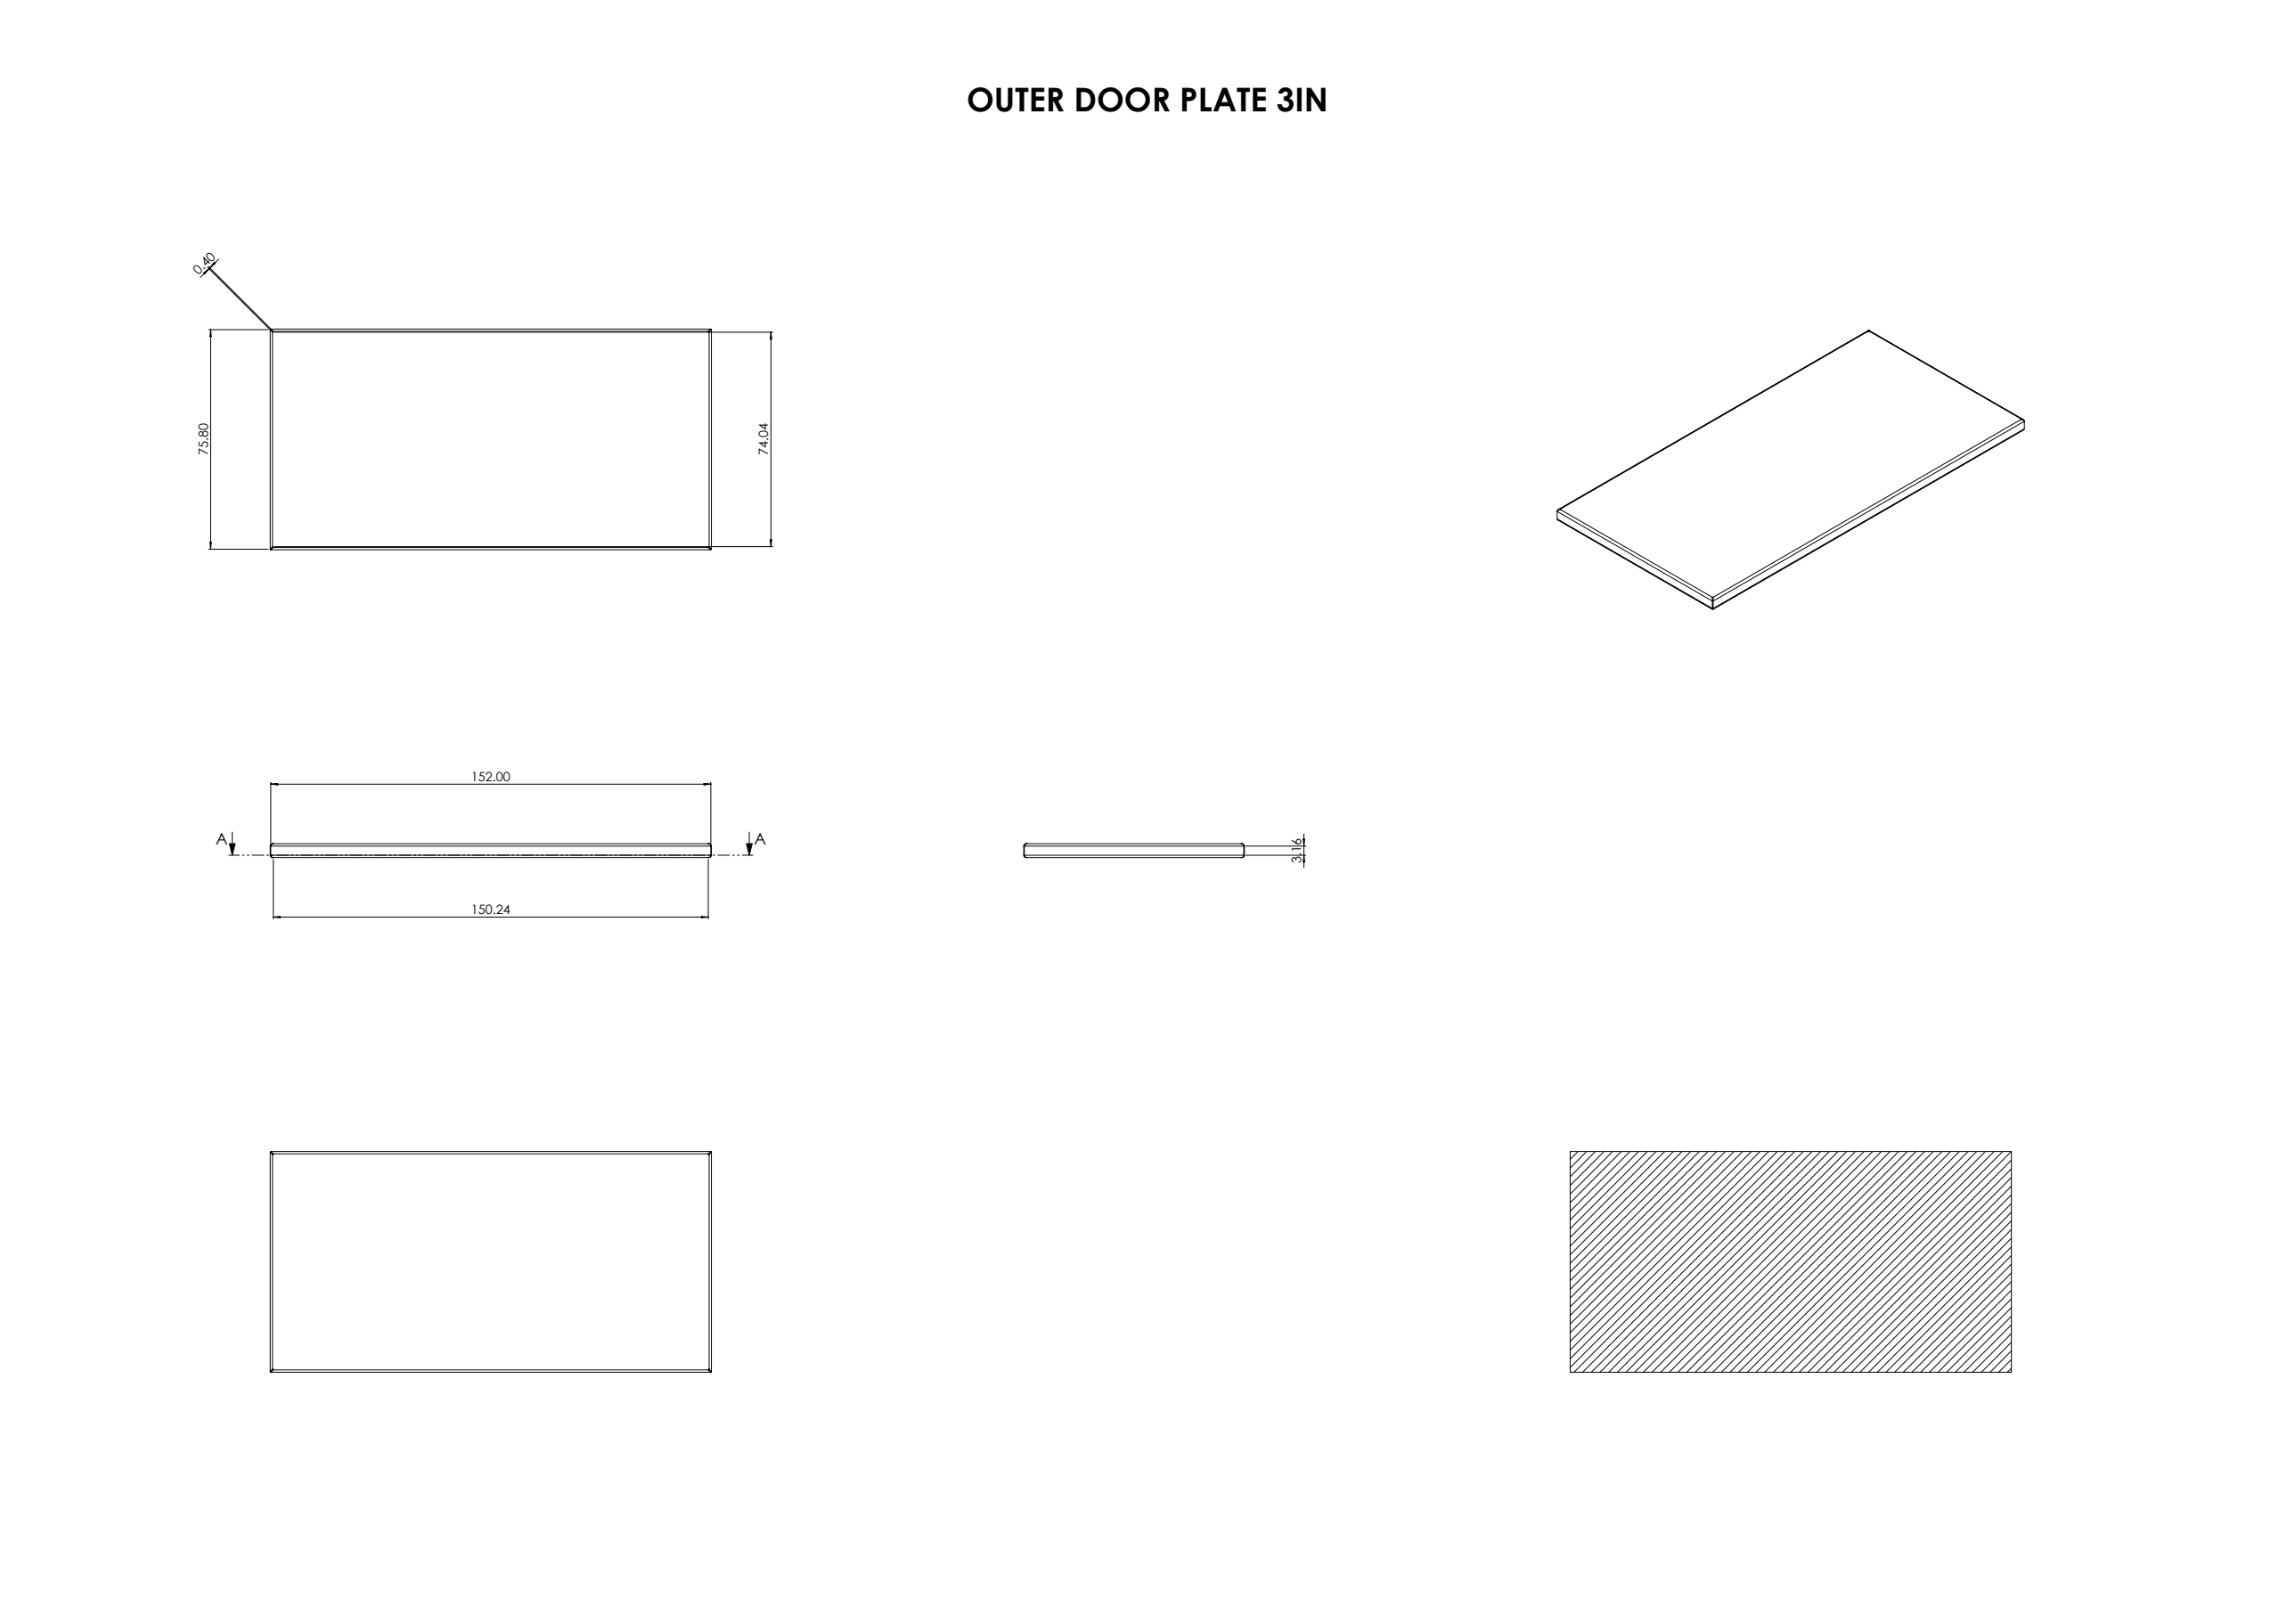
ISO-10303-21;
HEADER;
/* Generated by software containing ST-Developer
 * from STEP Tools, Inc. (www.steptools.com) 
 */

FILE_DESCRIPTION(
/* description */ (''),
/* implementation_level */ '2;1');

FILE_NAME(
/* name */ '03_Outer_Door_Plate_3in.step',
/* time_stamp */ '2026-10-25T01:30:15-07:00',
/* author */ (''),
/* organization */ (''),
/* preprocessor_version */ 'ST-DEVELOPER v20.2',
/* originating_system */ 'Autodesk Translation Framework v15.15.0.0',
/* authorisation */ '');

FILE_SCHEMA (('AUTOMOTIVE_DESIGN { 1 0 10303 214 3 1 1 }'));
ENDSEC;

DATA;
#10=MECHANICAL_DESIGN_GEOMETRIC_PRESENTATION_REPRESENTATION('',(#565),#32309);
#152=B_SPLINE_CURVE_WITH_KNOTS('',3,(#20657,#20658,#20659,#20660,#20661,
#20662,#20663,#20664,#20665,#20666,#20667,#20668,#20669,#20670,#20671,#20672,
#20673,#20674,#20675,#20676,#20677,#20678,#20679,#20680,#20681,#20682,#20683,
#20684,#20685,#20686,#20687,#20688,#20689,#20690,#20691,#20692,#20693,#20694,
#20695,#20696,#20697,#20698,#20699,#20700,#20701,#20702),.UNSPECIFIED.,
 .F.,.F.,(4,3,3,3,3,3,3,3,3,3,3,3,3,3,3,4),(0.,0.0572017311997787,0.120330894890366,
0.190833525217158,0.280000607595836,0.370000531646356,0.437396979142466,
0.498588004587218,0.56260087810271,0.634065239675333,0.727489847564673,
0.803842080660462,0.870326860442866,0.931777978459012,0.988871097354878,
1.),.UNSPECIFIED.);
#153=B_SPLINE_CURVE_WITH_KNOTS('',3,(#20704,#20705,#20706,#20707),
 .UNSPECIFIED.,.F.,.F.,(4,4),(0.,1.),.UNSPECIFIED.);
#154=B_SPLINE_CURVE_WITH_KNOTS('',3,(#20709,#20710,#20711,#20712,#20713,
#20714,#20715,#20716,#20717,#20718,#20719,#20720,#20721,#20722,#20723,#20724,
#20725,#20726,#20727,#20728,#20729,#20730,#20731,#20732,#20733,#20734,#20735,
#20736,#20737,#20738,#20739,#20740,#20741,#20742,#20743,#20744,#20745,#20746,
#20747,#20748,#20749,#20750,#20751,#20752,#20753,#20754),.UNSPECIFIED.,
 .F.,.F.,(4,3,3,3,3,3,3,3,3,3,3,3,3,3,3,4),(0.,0.0572030252319241,0.12033380234495,
0.190838689074404,0.28001183745251,0.370010357770946,0.43740667017455,0.498598114868611,
0.562610573399873,0.634075370124963,0.727505599815991,0.803852814389783,
0.870334971805663,0.931784146691265,0.988875797348581,1.),.UNSPECIFIED.);
#155=B_SPLINE_CURVE_WITH_KNOTS('',3,(#20782,#20783,#20784,#20785,#20786,
#20787,#20788,#20789,#20790,#20791,#20792,#20793,#20794,#20795,#20796,#20797,
#20798,#20799,#20800,#20801,#20802,#20803,#20804,#20805,#20806,#20807,#20808,
#20809,#20810,#20811,#20812,#20813,#20814,#20815,#20816,#20817,#20818,#20819,
#20820,#20821,#20822,#20823,#20824,#20825,#20826,#20827),.UNSPECIFIED.,
 .F.,.F.,(4,3,3,3,3,3,3,3,3,3,3,3,3,3,3,4),(0.,0.0572017311995356,0.120330894891212,
0.190833525222983,0.280000607602918,0.370000531652553,0.437396979149437,
0.498588004587769,0.562600878102254,0.634065239673979,0.727489847577867,
0.803842080671477,0.870326860452954,0.931777978465078,0.988871097360322,
1.),.UNSPECIFIED.);
#156=B_SPLINE_CURVE_WITH_KNOTS('',3,(#20829,#20830,#20831,#20832),
 .UNSPECIFIED.,.F.,.F.,(4,4),(0.,1.),.UNSPECIFIED.);
#157=B_SPLINE_CURVE_WITH_KNOTS('',3,(#20834,#20835,#20836,#20837,#20838,
#20839,#20840,#20841,#20842,#20843,#20844,#20845,#20846,#20847,#20848,#20849,
#20850,#20851,#20852,#20853,#20854,#20855,#20856,#20857,#20858,#20859,#20860,
#20861,#20862,#20863,#20864,#20865,#20866,#20867,#20868,#20869,#20870,#20871,
#20872,#20873,#20874,#20875,#20876,#20877,#20878,#20879),.UNSPECIFIED.,
 .F.,.F.,(4,3,3,3,3,3,3,3,3,3,3,3,3,3,3,4),(0.,0.0572030252292159,0.120333802342511,
0.190838689073324,0.280011837455233,0.370010357773329,0.437406670176794,
0.498598114483872,0.562610572991308,0.634075369653291,0.72750559895434,
0.803852813688791,0.870334971170512,0.931784146099022,0.988875796770373,
1.),.UNSPECIFIED.);
#158=B_SPLINE_CURVE_WITH_KNOTS('',3,(#20910,#20911,#20912,#20913,#20914,
#20915,#20916),.UNSPECIFIED.,.F.,.F.,(4,1,1,1,4),(-1.70953476876621,-1.22109626340444,
-0.732657758042664,-0.366328879021332,5.55111512312578E-17),
 .UNSPECIFIED.);
#159=B_SPLINE_CURVE_WITH_KNOTS('',3,(#20919,#20920,#20921,#20922,#20923,
#20924,#20925),.UNSPECIFIED.,.F.,.F.,(4,1,1,1,4),(-5.55111512312578E-17,
0.366328879021332,0.732657758042664,1.22109626340444,1.70953476876621),
 .UNSPECIFIED.);
#160=B_SPLINE_CURVE_WITH_KNOTS('',3,(#20956,#20957,#20958,#20959,#20960,
#20961),.UNSPECIFIED.,.F.,.F.,(4,1,1,4),(-1.70953476876627,-0.976877010723583,
-0.488438505361791,0.),.UNSPECIFIED.);
#161=B_SPLINE_CURVE_WITH_KNOTS('',3,(#20962,#20963,#20964,#20965,#20966,
#20967),.UNSPECIFIED.,.F.,.F.,(4,1,1,4),(0.,0.488438505361791,0.976877010723583,
1.70953476876627),.UNSPECIFIED.);
#162=B_SPLINE_CURVE_WITH_KNOTS('',3,(#20972,#20973,#20974,#20975,#20976,
#20977),.UNSPECIFIED.,.F.,.F.,(4,1,1,4),(-1.70953476876625,-0.976877010723563,
-0.48843850536177,2.22044604925036E-14),.UNSPECIFIED.);
#163=B_SPLINE_CURVE_WITH_KNOTS('',3,(#20979,#20980,#20981,#20982,#20983,
#20984,#20985,#20986,#20987,#20988,#20989,#20990,#20991,#20992,#20993,#20994,
#20995,#20996,#20997,#20998,#20999,#21000,#21001,#21002,#21003,#21004,#21005,
#21006,#21007,#21008,#21009,#21010,#21011,#21012,#21013,#21014,#21015,#21016,
#21017,#21018,#21019,#21020,#21021,#21022,#21023,#21024),.UNSPECIFIED.,
 .F.,.F.,(4,3,3,3,3,3,3,3,3,3,3,3,3,3,3,4),(0.,0.0572017312010985,0.120330894892007,
0.190833525228125,0.28000060761627,0.370000531664237,0.437396979166382,
0.498588004436113,0.562600877944707,0.634065239485818,0.727489847210369,
0.803842080370144,0.870326860183826,0.931777978218593,0.988871097121157,
1.),.UNSPECIFIED.);
#164=B_SPLINE_CURVE_WITH_KNOTS('',3,(#21034,#21035,#21036,#21037,#21038,
#21039,#21040,#21041,#21042,#21043,#21044,#21045,#21046,#21047,#21048,#21049,
#21050,#21051,#21052,#21053,#21054,#21055,#21056,#21057,#21058,#21059,#21060,
#21061,#21062,#21063,#21064,#21065,#21066,#21067,#21068,#21069,#21070,#21071,
#21072,#21073,#21074,#21075,#21076,#21077,#21078,#21079),.UNSPECIFIED.,
 .F.,.F.,(4,3,3,3,3,3,3,3,3,3,3,3,3,3,3,4),(0.,0.0572030252297135,0.120333802345235,
0.19083868907026,0.280011837447865,0.370010357766881,0.437406670170065,
0.498598115100775,0.562610573648761,0.634075370412809,0.727505600383724,
0.803852814849948,0.870334972221295,0.931784147083444,0.988875797723589,
1.),.UNSPECIFIED.);
#165=B_SPLINE_CURVE_WITH_KNOTS('',3,(#21080,#21081,#21082,#21083,#21084,
#21085),.UNSPECIFIED.,.F.,.F.,(4,1,1,4),(-2.2204460492503E-14,0.488438505361761,
0.976877010723545,1.70953476876622),.UNSPECIFIED.);
#166=B_SPLINE_CURVE_WITH_KNOTS('',3,(#21123,#21124,#21125,#21126),
 .UNSPECIFIED.,.F.,.F.,(4,4),(0.,1.),.UNSPECIFIED.);
#167=B_SPLINE_CURVE_WITH_KNOTS('',3,(#21128,#21129,#21130,#21131,#21132,
#21133,#21134,#21135,#21136,#21137,#21138,#21139,#21140,#21141,#21142,#21143,
#21144,#21145,#21146,#21147,#21148,#21149,#21150,#21151,#21152,#21153,#21154,
#21155,#21156,#21157,#21158,#21159,#21160,#21161,#21162,#21163,#21164,#21165,
#21166,#21167,#21168,#21169,#21170,#21171,#21172,#21173),.UNSPECIFIED.,
 .F.,.F.,(4,3,3,3,3,3,3,3,3,3,3,3,3,3,3,4),(0.,0.0572030252310299,0.120333802344518,
0.190838689075309,0.280011837457742,0.370010357775524,0.437406670179767,
0.498598114793286,0.562610573319674,0.634075370032691,0.727505599642952,
0.803852814249658,0.870334971678365,0.931784146571623,0.988875797229984,
1.),.UNSPECIFIED.);
#168=B_SPLINE_CURVE_WITH_KNOTS('',3,(#21200,#21201,#21202,#21203,#21204,
#21205,#21206,#21207,#21208,#21209,#21210,#21211,#21212,#21213,#21214,#21215,
#21216,#21217,#21218,#21219,#21220,#21221,#21222,#21223,#21224,#21225,#21226,
#21227,#21228,#21229,#21230,#21231,#21232,#21233,#21234,#21235,#21236,#21237,
#21238,#21239,#21240,#21241,#21242,#21243,#21244,#21245),.UNSPECIFIED.,
 .F.,.F.,(4,3,3,3,3,3,3,3,3,3,3,3,3,3,3,4),(0.,0.0572017311978579,0.120330894888584,
0.190833525218063,0.280000607593651,0.370000531644445,0.437396979144834,
0.498588004278573,0.562600877772937,0.634065239292226,0.727489846889499,
0.803842080110613,0.87032685994332,0.931777977987771,0.988871096896156,
1.),.UNSPECIFIED.);
#169=B_SPLINE_CURVE_WITH_KNOTS('',3,(#21246,#21247,#21248,#21249),
 .UNSPECIFIED.,.F.,.F.,(4,4),(0.,1.),.UNSPECIFIED.);
#170=B_SPLINE_CURVE_WITH_KNOTS('',3,(#21275,#21276,#21277,#21278,#21279,
#21280),.UNSPECIFIED.,.F.,.F.,(4,1,1,4),(-1.70953476876622,-0.976877010723545,
-0.488438505361761,2.2204460492503E-14),.UNSPECIFIED.);
#171=B_SPLINE_CURVE_WITH_KNOTS('',3,(#21310,#21311,#21312,#21313,#21314,
#21315),.UNSPECIFIED.,.F.,.F.,(4,1,1,4),(-2.22044604925036E-14,0.48843850536177,
0.976877010723563,1.70953476876625),.UNSPECIFIED.);
#172=B_SPLINE_CURVE_WITH_KNOTS('',3,(#21320,#21321,#21322,#21323,#21324,
#21325),.UNSPECIFIED.,.F.,.F.,(4,1,1,4),(-1.70953476876624,-0.976877010723568,
-0.488438505361784,0.),.UNSPECIFIED.);
#173=B_SPLINE_CURVE_WITH_KNOTS('',3,(#21327,#21328,#21329,#21330,#21331,
#21332,#21333,#21334,#21335,#21336,#21337,#21338,#21339,#21340,#21341,#21342,
#21343,#21344,#21345,#21346,#21347,#21348,#21349,#21350,#21351,#21352,#21353,
#21354,#21355,#21356,#21357,#21358,#21359,#21360,#21361,#21362,#21363,#21364,
#21365,#21366,#21367,#21368,#21369,#21370,#21371,#21372),.UNSPECIFIED.,
 .F.,.F.,(4,3,3,3,3,3,3,3,3,3,3,3,3,3,3,4),(0.,0.0572017312023357,0.120330894894396,
0.190833525223119,0.280000607603027,0.370000531652649,0.437396979148621,
0.498588004437818,0.562600877943201,0.634065239490927,0.727489847224149,
0.803842080384343,0.870326860191725,0.931777978222192,0.988871097126222,
1.),.UNSPECIFIED.);
#174=B_SPLINE_CURVE_WITH_KNOTS('',3,(#21380,#21381,#21382,#21383,#21384,
#21385,#21386,#21387,#21388,#21389,#21390,#21391,#21392,#21393,#21394,#21395,
#21396,#21397,#21398,#21399,#21400,#21401,#21402,#21403,#21404,#21405,#21406,
#21407,#21408,#21409,#21410,#21411,#21412,#21413,#21414,#21415,#21416,#21417,
#21418,#21419,#21420,#21421,#21422,#21423,#21424,#21425),.UNSPECIFIED.,
 .F.,.F.,(4,3,3,3,3,3,3,3,3,3,3,3,3,3,3,4),(0.,0.0572030252293332,0.120333802342866,
0.190838689071281,0.280011837454217,0.37001035777244,0.437406670175742,
0.498598114943859,0.562610573478433,0.634075370216571,0.727505599976586,
0.803852814520644,0.870334971919668,0.93178414679375,0.988875797446903,
1.),.UNSPECIFIED.);
#175=B_SPLINE_CURVE_WITH_KNOTS('',3,(#21426,#21427,#21428,#21429,#21430,
#21431),.UNSPECIFIED.,.F.,.F.,(4,1,1,4),(0.,0.488438505361779,0.976877010723558,
1.70953476876623),.UNSPECIFIED.);
#176=B_SPLINE_CURVE_WITH_KNOTS('',3,(#21457,#21458,#21459,#21460,#21461,
#21462,#21463,#21464,#21465,#21466,#21467,#21468,#21469,#21470,#21471,#21472,
#21473,#21474,#21475,#21476,#21477,#21478,#21479,#21480,#21481,#21482,#21483,
#21484,#21485,#21486,#21487,#21488,#21489,#21490,#21491,#21492,#21493,#21494,
#21495,#21496,#21497,#21498,#21499,#21500,#21501,#21502),.UNSPECIFIED.,
 .F.,.F.,(4,3,3,3,3,3,3,3,3,3,3,3,3,3,3,4),(0.,0.0572017311998059,0.120330894890615,
0.190833525219348,0.280000607590358,0.370000531641563,0.437396979142138,
0.498588004431166,0.562600877935177,0.634065239482274,0.72748984722562,
0.803842080384528,0.870326860191735,0.931777978221736,0.988871097122214,
1.),.UNSPECIFIED.);
#177=B_SPLINE_CURVE_WITH_KNOTS('',3,(#21503,#21504,#21505,#21506),
 .UNSPECIFIED.,.F.,.F.,(4,4),(0.,1.),.UNSPECIFIED.);
#178=B_SPLINE_CURVE_WITH_KNOTS('',3,(#21532,#21533,#21534,#21535),
 .UNSPECIFIED.,.F.,.F.,(4,4),(0.,1.),.UNSPECIFIED.);
#179=B_SPLINE_CURVE_WITH_KNOTS('',3,(#21537,#21538,#21539,#21540,#21541,
#21542,#21543,#21544,#21545,#21546,#21547,#21548,#21549,#21550,#21551,#21552,
#21553,#21554,#21555,#21556,#21557,#21558,#21559,#21560,#21561,#21562,#21563,
#21564,#21565,#21566,#21567,#21568,#21569,#21570,#21571,#21572,#21573,#21574,
#21575,#21576,#21577,#21578,#21579,#21580,#21581,#21582),.UNSPECIFIED.,
 .F.,.F.,(4,3,3,3,3,3,3,3,3,3,3,3,3,3,3,4),(0.,0.0572030252325847,0.120333802345704,
0.190838689075859,0.280011837455415,0.370010357773488,0.437406670178867,
0.498598114640677,0.562610573158014,0.634075369846179,0.727505599307959,
0.803852813976729,0.870334971429114,0.931784146336173,0.98887579700217,
1.),.UNSPECIFIED.);
#180=B_SPLINE_CURVE_WITH_KNOTS('',3,(#21610,#21611,#21612,#21613,#21614,
#21615),.UNSPECIFIED.,.F.,.F.,(4,1,1,4),(0.,0.488438505361784,0.976877010723568,
1.70953476876624),.UNSPECIFIED.);
#181=B_SPLINE_CURVE_WITH_KNOTS('',3,(#21644,#21645,#21646,#21647,#21648,
#21649),.UNSPECIFIED.,.F.,.F.,(4,1,1,4),(-1.70953476876623,-0.976877010723558,
-0.488438505361779,0.),.UNSPECIFIED.);
#182=B_SPLINE_CURVE_WITH_KNOTS('',3,(#21675,#21676,#21677,#21678,#21679,
#21680,#21681,#21682,#21683,#21684,#21685,#21686,#21687,#21688,#21689,#21690,
#21691,#21692,#21693,#21694,#21695,#21696,#21697,#21698,#21699,#21700,#21701,
#21702,#21703,#21704,#21705,#21706,#21707,#21708,#21709,#21710,#21711,#21712,
#21713,#21714,#21715,#21716,#21717,#21718,#21719,#21720),.UNSPECIFIED.,
 .F.,.F.,(4,3,3,3,3,3,3,3,3,3,3,3,3,3,3,4),(0.,0.0572017311990066,0.12033089488981,
0.190833525218569,0.280000607592288,0.370000531643252,0.437396979144409,
0.498588004504094,0.562600878013463,0.634065239570545,0.727489847383163,
0.803842080513076,0.87032686030984,0.931777978330153,0.988871097227407,
1.),.UNSPECIFIED.);
#183=B_SPLINE_CURVE_WITH_KNOTS('',3,(#21722,#21723,#21724,#21725),
 .UNSPECIFIED.,.F.,.F.,(4,4),(-1.,0.),.UNSPECIFIED.);
#184=B_SPLINE_CURVE_WITH_KNOTS('',3,(#21726,#21727,#21728,#21729,#21730,
#21731,#21732,#21733,#21734,#21735,#21736,#21737,#21738,#21739,#21740,#21741,
#21742,#21743,#21744,#21745,#21746,#21747,#21748,#21749,#21750,#21751,#21752,
#21753,#21754,#21755,#21756,#21757,#21758,#21759,#21760,#21761,#21762,#21763,
#21764,#21765,#21766,#21767,#21768,#21769,#21770,#21771),.UNSPECIFIED.,
 .F.,.F.,(4,3,3,3,3,3,3,3,3,3,3,3,3,3,3,4),(0.,0.0572030252278138,0.120333802343175,
0.190838689074842,0.280011837442225,0.370010357761947,0.437406670170392,
0.498598115021839,0.562610573562917,0.634075370316736,0.727505600127926,
0.803852814646169,0.87033497203609,0.931784146912104,0.988875797559871,
1.),.UNSPECIFIED.);
#185=B_SPLINE_CURVE_WITH_KNOTS('',3,(#21798,#21799,#21800,#21801,#21802,
#21803,#21804,#21805,#21806,#21807,#21808,#21809,#21810,#21811,#21812,#21813,
#21814,#21815,#21816,#21817,#21818,#21819,#21820,#21821,#21822,#21823,#21824,
#21825,#21826,#21827,#21828,#21829,#21830,#21831,#21832,#21833,#21834,#21835,
#21836,#21837,#21838,#21839,#21840,#21841,#21842,#21843),.UNSPECIFIED.,
 .F.,.F.,(4,3,3,3,3,3,3,3,3,3,3,3,3,3,3,4),(0.,0.0572017312051678,0.12033089489696,
0.190833525228863,0.280000607608025,0.370000531657022,0.437396979162787,
0.498588004452882,0.562600877959885,0.63406523951468,0.727489847284879,
0.803842080435825,0.870326860243776,0.93177797826367,0.988871097172671,
1.),.UNSPECIFIED.);
#186=B_SPLINE_CURVE_WITH_KNOTS('',3,(#21845,#21846,#21847,#21848),
 .UNSPECIFIED.,.F.,.F.,(4,4),(0.,1.),.UNSPECIFIED.);
#187=B_SPLINE_CURVE_WITH_KNOTS('',3,(#21850,#21851,#21852,#21853,#21854,
#21855,#21856,#21857,#21858,#21859,#21860,#21861,#21862,#21863,#21864,#21865,
#21866,#21867,#21868,#21869,#21870,#21871,#21872,#21873,#21874,#21875,#21876,
#21877,#21878,#21879,#21880,#21881,#21882,#21883,#21884,#21885,#21886,#21887,
#21888,#21889,#21890,#21891,#21892,#21893,#21894,#21895),.UNSPECIFIED.,
 .F.,.F.,(4,3,3,3,3,3,3,3,3,3,3,3,3,3,3,4),(0.,0.0572030252315006,0.120333802344992,
0.190838689075267,0.280011837456553,0.370010357774484,0.437406670177093,
0.498598114715166,0.562610573236497,0.634075369937252,0.727505599475578,
0.803852814112987,0.870334971553103,0.931784146452336,0.988875797114711,
1.),.UNSPECIFIED.);
#188=B_SPLINE_CURVE_WITH_KNOTS('',3,(#21922,#21923,#21924,#21925,#21926,
#21927),.UNSPECIFIED.,.F.,.F.,(4,1,1,4),(-1.7095347687662,-0.97687701072354,
-0.488438505361764,1.11854969730985E-14),.UNSPECIFIED.);
#189=B_SPLINE_CURVE_WITH_KNOTS('',3,(#21930,#21931,#21932,#21933,#21934,
#21935),.UNSPECIFIED.,.F.,.F.,(4,1,1,4),(-1.11854969730985E-14,0.488438505361764,
0.97687701072354,1.7095347687662),.UNSPECIFIED.);
#190=B_SPLINE_CURVE_WITH_KNOTS('',3,(#21966,#21967,#21968,#21969,#21970,
#21971),.UNSPECIFIED.,.F.,.F.,(4,1,1,4),(1.43205788482356,2.16471564286623,
2.65315414822802,3.1415926535898),.UNSPECIFIED.);
#191=B_SPLINE_CURVE_WITH_KNOTS('',3,(#21972,#21973,#21974,#21975,#21976,
#21977),.UNSPECIFIED.,.F.,.F.,(4,1,1,4),(-3.1415926535898,-2.65315414822802,
-2.16471564286623,-1.43205788482356),.UNSPECIFIED.);
#431=B_SPLINE_SURFACE_WITH_KNOTS('',3,3,((#20631,#20632,#20633,#20634,#20635,
#20636),(#20637,#20638,#20639,#20640,#20641,#20642),(#20643,#20644,#20645,
#20646,#20647,#20648),(#20649,#20650,#20651,#20652,#20653,#20654)),
 .UNSPECIFIED.,.F.,.F.,.F.,(4,4),(4,1,1,4),(0.,1.),(0.,0.571428571428571,
0.857142857142857,1.),.UNSPECIFIED.);
#432=B_SPLINE_SURFACE_WITH_KNOTS('',3,3,((#20756,#20757,#20758,#20759,#20760,
#20761),(#20762,#20763,#20764,#20765,#20766,#20767),(#20768,#20769,#20770,
#20771,#20772,#20773),(#20774,#20775,#20776,#20777,#20778,#20779)),
 .UNSPECIFIED.,.F.,.F.,.F.,(4,4),(4,1,1,4),(0.,1.),(0.,0.571428571428571,
0.857142857142857,1.),.UNSPECIFIED.);
#433=B_SPLINE_SURFACE_WITH_KNOTS('',3,3,((#20881,#20882,#20883,#20884,#20885,
#20886,#20887),(#20888,#20889,#20890,#20891,#20892,#20893,#20894),(#20895,
#20896,#20897,#20898,#20899,#20900,#20901),(#20902,#20903,#20904,#20905,
#20906,#20907,#20908)),.UNSPECIFIED.,.F.,.F.,.F.,(4,4),(4,1,1,1,4),(0.,
1.),(-1.70953476876621,-1.22109626340444,-0.732657758042664,-0.366328879021332,
5.55111512312578E-17),.UNSPECIFIED.);
#434=B_SPLINE_SURFACE_WITH_KNOTS('',3,3,((#20932,#20933,#20934,#20935,#20936,
#20937),(#20938,#20939,#20940,#20941,#20942,#20943),(#20944,#20945,#20946,
#20947,#20948,#20949),(#20950,#20951,#20952,#20953,#20954,#20955)),
 .UNSPECIFIED.,.F.,.F.,.F.,(4,4),(4,1,1,4),(0.,1.),(-1.70953476876627,-0.976877010723583,
-0.488438505361791,0.),.UNSPECIFIED.);
#435=B_SPLINE_SURFACE_WITH_KNOTS('',3,3,((#21098,#21099,#21100,#21101,#21102,
#21103),(#21104,#21105,#21106,#21107,#21108,#21109),(#21110,#21111,#21112,
#21113,#21114,#21115),(#21116,#21117,#21118,#21119,#21120,#21121)),
 .UNSPECIFIED.,.F.,.F.,.F.,(4,4),(4,1,1,4),(0.,1.),(0.,0.571428571428571,
0.857142857142857,1.),.UNSPECIFIED.);
#436=B_SPLINE_SURFACE_WITH_KNOTS('',3,3,((#21175,#21176,#21177,#21178,#21179,
#21180),(#21181,#21182,#21183,#21184,#21185,#21186),(#21187,#21188,#21189,
#21190,#21191,#21192),(#21193,#21194,#21195,#21196,#21197,#21198)),
 .UNSPECIFIED.,.F.,.F.,.F.,(4,4),(4,1,1,4),(0.,1.),(0.,0.571428571428571,
0.857142857142857,1.),.UNSPECIFIED.);
#437=B_SPLINE_SURFACE_WITH_KNOTS('',3,3,((#21250,#21251,#21252,#21253,#21254,
#21255),(#21256,#21257,#21258,#21259,#21260,#21261),(#21262,#21263,#21264,
#21265,#21266,#21267),(#21268,#21269,#21270,#21271,#21272,#21273)),
 .UNSPECIFIED.,.F.,.F.,.F.,(4,4),(4,1,1,4),(0.,1.),(-1.70953476876622,-0.976877010723545,
-0.488438505361761,2.2204460492503E-14),.UNSPECIFIED.);
#438=B_SPLINE_SURFACE_WITH_KNOTS('',3,3,((#21286,#21287,#21288,#21289,#21290,
#21291),(#21292,#21293,#21294,#21295,#21296,#21297),(#21298,#21299,#21300,
#21301,#21302,#21303),(#21304,#21305,#21306,#21307,#21308,#21309)),
 .UNSPECIFIED.,.F.,.F.,.F.,(4,4),(4,1,1,4),(0.,1.),(-1.70953476876625,-0.976877010723563,
-0.48843850536177,2.22044604925036E-14),.UNSPECIFIED.);
#439=B_SPLINE_SURFACE_WITH_KNOTS('',3,3,((#21432,#21433,#21434,#21435,#21436,
#21437),(#21438,#21439,#21440,#21441,#21442,#21443),(#21444,#21445,#21446,
#21447,#21448,#21449),(#21450,#21451,#21452,#21453,#21454,#21455)),
 .UNSPECIFIED.,.F.,.F.,.F.,(4,4),(4,1,1,4),(0.,1.),(0.,0.571428571428571,
0.857142857142857,1.),.UNSPECIFIED.);
#440=B_SPLINE_SURFACE_WITH_KNOTS('',3,3,((#21507,#21508,#21509,#21510,#21511,
#21512),(#21513,#21514,#21515,#21516,#21517,#21518),(#21519,#21520,#21521,
#21522,#21523,#21524),(#21525,#21526,#21527,#21528,#21529,#21530)),
 .UNSPECIFIED.,.F.,.F.,.F.,(4,4),(4,1,1,4),(0.,1.),(0.,0.571428571428571,
0.857142857142857,1.),.UNSPECIFIED.);
#441=B_SPLINE_SURFACE_WITH_KNOTS('',3,3,((#21584,#21585,#21586,#21587,#21588,
#21589),(#21590,#21591,#21592,#21593,#21594,#21595),(#21596,#21597,#21598,
#21599,#21600,#21601),(#21602,#21603,#21604,#21605,#21606,#21607)),
 .UNSPECIFIED.,.F.,.F.,.F.,(4,4),(4,1,1,4),(0.,1.),(-1.70953476876624,-0.976877010723568,
-0.488438505361784,0.),.UNSPECIFIED.);
#442=B_SPLINE_SURFACE_WITH_KNOTS('',3,3,((#21620,#21621,#21622,#21623,#21624,
#21625),(#21626,#21627,#21628,#21629,#21630,#21631),(#21632,#21633,#21634,
#21635,#21636,#21637),(#21638,#21639,#21640,#21641,#21642,#21643)),
 .UNSPECIFIED.,.F.,.F.,.F.,(4,4),(4,1,1,4),(0.,1.),(-1.70953476876623,-0.976877010723558,
-0.488438505361779,0.),.UNSPECIFIED.);
#443=B_SPLINE_SURFACE_WITH_KNOTS('',3,3,((#21650,#21651,#21652,#21653,#21654,
#21655),(#21656,#21657,#21658,#21659,#21660,#21661),(#21662,#21663,#21664,
#21665,#21666,#21667),(#21668,#21669,#21670,#21671,#21672,#21673)),
 .UNSPECIFIED.,.F.,.F.,.F.,(4,4),(4,1,1,4),(0.,1.),(0.,0.571428571428571,
0.857142857142857,1.),.UNSPECIFIED.);
#444=B_SPLINE_SURFACE_WITH_KNOTS('',3,3,((#21772,#21773,#21774,#21775,#21776,
#21777),(#21778,#21779,#21780,#21781,#21782,#21783),(#21784,#21785,#21786,
#21787,#21788,#21789),(#21790,#21791,#21792,#21793,#21794,#21795)),
 .UNSPECIFIED.,.F.,.F.,.F.,(4,4),(4,1,1,4),(0.,1.),(0.,0.571428571428571,
0.857142857142857,1.),.UNSPECIFIED.);
#445=B_SPLINE_SURFACE_WITH_KNOTS('',3,3,((#21897,#21898,#21899,#21900,#21901,
#21902),(#21903,#21904,#21905,#21906,#21907,#21908),(#21909,#21910,#21911,
#21912,#21913,#21914),(#21915,#21916,#21917,#21918,#21919,#21920)),
 .UNSPECIFIED.,.F.,.F.,.F.,(4,4),(4,1,1,4),(0.,1.),(-1.7095347687662,-0.97687701072354,
-0.488438505361764,1.11854969730985E-14),.UNSPECIFIED.);
#446=B_SPLINE_SURFACE_WITH_KNOTS('',3,3,((#21942,#21943,#21944,#21945,#21946,
#21947),(#21948,#21949,#21950,#21951,#21952,#21953),(#21954,#21955,#21956,
#21957,#21958,#21959),(#21960,#21961,#21962,#21963,#21964,#21965)),
 .UNSPECIFIED.,.F.,.F.,.F.,(4,4),(4,1,1,4),(0.,1.),(-3.1415926535898,-2.65315414822802,
-2.16471564286623,-1.43205788482356),.UNSPECIFIED.);
#537=SHAPE_REPRESENTATION_RELATIONSHIP('SRR','None',#32364,#551);
#551=ADVANCED_BREP_SHAPE_REPRESENTATION('',(#579),#32297);
#565=STYLED_ITEM('',(#32495),#579);
#579=MANIFOLD_SOLID_BREP('Body1',#13806);
#668=CYLINDRICAL_SURFACE('',#14097,0.8);
#669=CYLINDRICAL_SURFACE('',#14099,0.8);
#670=CYLINDRICAL_SURFACE('',#14102,0.8);
#671=CYLINDRICAL_SURFACE('',#14104,0.8);
#672=CYLINDRICAL_SURFACE('',#14107,0.8);
#673=CYLINDRICAL_SURFACE('',#14109,0.8);
#674=CYLINDRICAL_SURFACE('',#14110,0.8);
#675=CYLINDRICAL_SURFACE('',#14112,0.8);
#1339=FACE_OUTER_BOUND('',#2142,.T.);
#1340=FACE_OUTER_BOUND('',#2143,.T.);
#1341=FACE_OUTER_BOUND('',#2144,.T.);
#1342=FACE_OUTER_BOUND('',#2145,.T.);
#1343=FACE_OUTER_BOUND('',#2146,.T.);
#1344=FACE_OUTER_BOUND('',#2147,.T.);
#1345=FACE_OUTER_BOUND('',#2148,.T.);
#1346=FACE_OUTER_BOUND('',#2149,.T.);
#1347=FACE_OUTER_BOUND('',#2150,.T.);
#1348=FACE_OUTER_BOUND('',#2151,.T.);
#1349=FACE_OUTER_BOUND('',#2152,.T.);
#1350=FACE_OUTER_BOUND('',#2153,.T.);
#1351=FACE_OUTER_BOUND('',#2154,.T.);
#1352=FACE_OUTER_BOUND('',#2155,.T.);
#1353=FACE_OUTER_BOUND('',#2156,.T.);
#1354=FACE_OUTER_BOUND('',#2157,.T.);
#1355=FACE_OUTER_BOUND('',#2158,.T.);
#1356=FACE_OUTER_BOUND('',#2159,.T.);
#1357=FACE_OUTER_BOUND('',#2160,.T.);
#1358=FACE_OUTER_BOUND('',#2161,.T.);
#1359=FACE_OUTER_BOUND('',#2162,.T.);
#1360=FACE_OUTER_BOUND('',#2163,.T.);
#1361=FACE_OUTER_BOUND('',#2164,.T.);
#1362=FACE_OUTER_BOUND('',#2165,.T.);
#1363=FACE_OUTER_BOUND('',#2166,.T.);
#1364=FACE_OUTER_BOUND('',#2167,.T.);
#1365=FACE_OUTER_BOUND('',#2168,.T.);
#1366=FACE_OUTER_BOUND('',#2169,.T.);
#1367=FACE_OUTER_BOUND('',#2170,.T.);
#1368=FACE_OUTER_BOUND('',#2171,.T.);
#1369=FACE_OUTER_BOUND('',#2172,.T.);
#1370=FACE_OUTER_BOUND('',#2173,.T.);
#1371=FACE_OUTER_BOUND('',#2174,.T.);
#1372=FACE_OUTER_BOUND('',#2175,.T.);
#2142=EDGE_LOOP('',(#9157,#9158,#9159,#9160));
#2143=EDGE_LOOP('',(#9161,#9162,#9163,#9164));
#2144=EDGE_LOOP('',(#9165,#9166,#9167,#9168));
#2145=EDGE_LOOP('',(#9169,#9170,#9171,#9172));
#2146=EDGE_LOOP('',(#9173,#9174,#9175,#9176));
#2147=EDGE_LOOP('',(#9177,#9178,#9179,#9180,#9181,#9182));
#2148=EDGE_LOOP('',(#9183,#9184,#9185,#9186));
#2149=EDGE_LOOP('',(#9187,#9188,#9189,#9190,#9191,#9192));
#2150=EDGE_LOOP('',(#9193,#9194,#9195,#9196,#9197,#9198,#9199,#9200));
#2151=EDGE_LOOP('',(#9201,#9202,#9203,#9204));
#2152=EDGE_LOOP('',(#9205,#9206,#9207,#9208));
#2153=EDGE_LOOP('',(#9209,#9210,#9211,#9212));
#2154=EDGE_LOOP('',(#9213,#9214,#9215,#9216));
#2155=EDGE_LOOP('',(#9217,#9218,#9219,#9220));
#2156=EDGE_LOOP('',(#9221,#9222,#9223,#9224,#9225,#9226));
#2157=EDGE_LOOP('',(#9227,#9228,#9229,#9230));
#2158=EDGE_LOOP('',(#9231,#9232,#9233,#9234,#9235,#9236));
#2159=EDGE_LOOP('',(#9237,#9238,#9239,#9240));
#2160=EDGE_LOOP('',(#9241,#9242,#9243,#9244));
#2161=EDGE_LOOP('',(#9245,#9246,#9247,#9248));
#2162=EDGE_LOOP('',(#9249,#9250,#9251,#9252));
#2163=EDGE_LOOP('',(#9253,#9254,#9255,#9256));
#2164=EDGE_LOOP('',(#9257,#9258,#9259,#9260));
#2165=EDGE_LOOP('',(#9261,#9262,#9263,#9264));
#2166=EDGE_LOOP('',(#9265,#9266,#9267,#9268));
#2167=EDGE_LOOP('',(#9269,#9270,#9271,#9272));
#2168=EDGE_LOOP('',(#9273,#9274,#9275,#9276));
#2169=EDGE_LOOP('',(#9277,#9278,#9279,#9280,#9281,#9282));
#2170=EDGE_LOOP('',(#9283,#9284,#9285,#9286));
#2171=EDGE_LOOP('',(#9287,#9288,#9289,#9290,#9291,#9292));
#2172=EDGE_LOOP('',(#9293,#9294,#9295,#9296,#9297,#9298));
#2173=EDGE_LOOP('',(#9299,#9300,#9301,#9302,#9303,#9304,#9305,#9306));
#2174=EDGE_LOOP('',(#9307,#9308,#9309,#9310,#9311,#9312));
#2175=EDGE_LOOP('',(#9313,#9314,#9315,#9316));
#3025=LINE('',#20755,#4336);
#3026=LINE('',#20880,#4337);
#3027=LINE('',#20918,#4338);
#3028=LINE('',#20929,#4339);
#3029=LINE('',#20930,#4340);
#3030=LINE('',#20931,#4341);
#3031=LINE('',#20970,#4342);
#3032=LINE('',#21025,#4343);
#3033=LINE('',#21028,#4344);
#3034=LINE('',#21029,#4345);
#3035=LINE('',#21032,#4346);
#3036=LINE('',#21088,#4347);
#3037=LINE('',#21090,#4348);
#3038=LINE('',#21092,#4349);
#3039=LINE('',#21094,#4350);
#3040=LINE('',#21096,#4351);
#3041=LINE('',#21097,#4352);
#3042=LINE('',#21174,#4353);
#3043=LINE('',#21281,#4354);
#3044=LINE('',#21284,#4355);
#3045=LINE('',#21285,#4356);
#3046=LINE('',#21318,#4357);
#3047=LINE('',#21373,#4358);
#3048=LINE('',#21376,#4359);
#3049=LINE('',#21377,#4360);
#3050=LINE('',#21583,#4361);
#3051=LINE('',#21609,#4362);
#3052=LINE('',#21618,#4363);
#3053=LINE('',#21619,#4364);
#3054=LINE('',#21896,#4365);
#3055=LINE('',#21929,#4366);
#3056=LINE('',#21938,#4367);
#3057=LINE('',#21940,#4368);
#3058=LINE('',#21941,#4369);
#3059=LINE('',#21979,#4370);
#3060=LINE('',#21981,#4371);
#3061=LINE('',#21983,#4372);
#3062=LINE('',#21985,#4373);
#3063=LINE('',#21986,#4374);
#3064=LINE('',#21989,#4375);
#4336=VECTOR('',#15379,10.);
#4337=VECTOR('',#15380,10.);
#4338=VECTOR('',#15381,10.);
#4339=VECTOR('',#15384,10.);
#4340=VECTOR('',#15385,10.);
#4341=VECTOR('',#15386,10.);
#4342=VECTOR('',#15389,10.);
#4343=VECTOR('',#15390,10.);
#4344=VECTOR('',#15393,10.);
#4345=VECTOR('',#15394,10.);
#4346=VECTOR('',#15397,10.);
#4347=VECTOR('',#15400,10.);
#4348=VECTOR('',#15401,10.);
#4349=VECTOR('',#15402,10.);
#4350=VECTOR('',#15403,10.);
#4351=VECTOR('',#15404,10.);
#4352=VECTOR('',#15405,10.);
#4353=VECTOR('',#15406,10.);
#4354=VECTOR('',#15407,10.);
#4355=VECTOR('',#15410,10.);
#4356=VECTOR('',#15411,10.);
#4357=VECTOR('',#15414,10.);
#4358=VECTOR('',#15415,10.);
#4359=VECTOR('',#15418,10.);
#4360=VECTOR('',#15419,10.);
#4361=VECTOR('',#15422,10.);
#4362=VECTOR('',#15423,10.);
#4363=VECTOR('',#15426,10.);
#4364=VECTOR('',#15427,10.);
#4365=VECTOR('',#15428,10.);
#4366=VECTOR('',#15429,10.);
#4367=VECTOR('',#15432,10.);
#4368=VECTOR('',#15433,10.);
#4369=VECTOR('',#15434,10.);
#4370=VECTOR('',#15437,10.);
#4371=VECTOR('',#15440,10.);
#4372=VECTOR('',#15443,10.);
#4373=VECTOR('',#15446,10.);
#4374=VECTOR('',#15447,10.);
#4375=VECTOR('',#15452,10.);
#5664=VERTEX_POINT('',#20655);
#5665=VERTEX_POINT('',#20656);
#5666=VERTEX_POINT('',#20703);
#5667=VERTEX_POINT('',#20708);
#5668=VERTEX_POINT('',#20780);
#5669=VERTEX_POINT('',#20781);
#5670=VERTEX_POINT('',#20828);
#5671=VERTEX_POINT('',#20833);
#5672=VERTEX_POINT('',#20909);
#5673=VERTEX_POINT('',#20917);
#5674=VERTEX_POINT('',#20927);
#5675=VERTEX_POINT('',#20928);
#5676=VERTEX_POINT('',#20969);
#5677=VERTEX_POINT('',#20971);
#5678=VERTEX_POINT('',#20978);
#5679=VERTEX_POINT('',#21027);
#5680=VERTEX_POINT('',#21031);
#5681=VERTEX_POINT('',#21033);
#5682=VERTEX_POINT('',#21087);
#5683=VERTEX_POINT('',#21089);
#5684=VERTEX_POINT('',#21091);
#5685=VERTEX_POINT('',#21093);
#5686=VERTEX_POINT('',#21095);
#5687=VERTEX_POINT('',#21122);
#5688=VERTEX_POINT('',#21127);
#5689=VERTEX_POINT('',#21199);
#5690=VERTEX_POINT('',#21274);
#5691=VERTEX_POINT('',#21283);
#5692=VERTEX_POINT('',#21317);
#5693=VERTEX_POINT('',#21319);
#5694=VERTEX_POINT('',#21326);
#5695=VERTEX_POINT('',#21375);
#5696=VERTEX_POINT('',#21379);
#5697=VERTEX_POINT('',#21456);
#5698=VERTEX_POINT('',#21531);
#5699=VERTEX_POINT('',#21536);
#5700=VERTEX_POINT('',#21608);
#5701=VERTEX_POINT('',#21617);
#5702=VERTEX_POINT('',#21674);
#5703=VERTEX_POINT('',#21721);
#5704=VERTEX_POINT('',#21796);
#5705=VERTEX_POINT('',#21797);
#5706=VERTEX_POINT('',#21844);
#5707=VERTEX_POINT('',#21849);
#5708=VERTEX_POINT('',#21921);
#5709=VERTEX_POINT('',#21928);
#5710=VERTEX_POINT('',#21937);
#5711=VERTEX_POINT('',#21939);
#6955=EDGE_CURVE('',#5664,#5665,#152,.T.);
#6956=EDGE_CURVE('',#5666,#5665,#153,.T.);
#6957=EDGE_CURVE('',#5666,#5667,#154,.T.);
#6958=EDGE_CURVE('',#5667,#5664,#3025,.T.);
#6959=EDGE_CURVE('',#5668,#5669,#155,.T.);
#6960=EDGE_CURVE('',#5670,#5669,#156,.T.);
#6961=EDGE_CURVE('',#5670,#5671,#157,.T.);
#6962=EDGE_CURVE('',#5671,#5668,#3026,.T.);
#6963=EDGE_CURVE('',#5669,#5672,#158,.T.);
#6964=EDGE_CURVE('',#5672,#5673,#3027,.T.);
#6965=EDGE_CURVE('',#5673,#5670,#159,.T.);
#6966=EDGE_CURVE('',#5674,#5675,#3028,.T.);
#6967=EDGE_CURVE('',#5675,#5673,#3029,.T.);
#6968=EDGE_CURVE('',#5672,#5674,#3030,.T.);
#6969=EDGE_CURVE('',#5665,#5675,#160,.T.);
#6970=EDGE_CURVE('',#5674,#5666,#161,.T.);
#6971=EDGE_CURVE('',#5674,#5676,#3031,.T.);
#6972=EDGE_CURVE('',#5677,#5676,#162,.T.);
#6973=EDGE_CURVE('',#5678,#5677,#163,.T.);
#6974=EDGE_CURVE('',#5678,#5667,#3032,.T.);
#6975=EDGE_CURVE('',#5679,#5672,#3033,.T.);
#6976=EDGE_CURVE('',#5676,#5679,#3034,.T.);
#6977=EDGE_CURVE('',#5668,#5680,#3035,.T.);
#6978=EDGE_CURVE('',#5681,#5680,#164,.T.);
#6979=EDGE_CURVE('',#5679,#5681,#165,.T.);
#6980=EDGE_CURVE('',#5682,#5671,#3036,.T.);
#6981=EDGE_CURVE('',#5683,#5682,#3037,.T.);
#6982=EDGE_CURVE('',#5684,#5683,#3038,.T.);
#6983=EDGE_CURVE('',#5685,#5684,#3039,.T.);
#6984=EDGE_CURVE('',#5686,#5685,#3040,.T.);
#6985=EDGE_CURVE('',#5680,#5686,#3041,.T.);
#6986=EDGE_CURVE('',#5687,#5677,#166,.T.);
#6987=EDGE_CURVE('',#5687,#5688,#167,.T.);
#6988=EDGE_CURVE('',#5688,#5678,#3042,.T.);
#6989=EDGE_CURVE('',#5686,#5689,#168,.T.);
#6990=EDGE_CURVE('',#5681,#5689,#169,.T.);
#6991=EDGE_CURVE('',#5689,#5690,#170,.T.);
#6992=EDGE_CURVE('',#5690,#5679,#3043,.T.);
#6993=EDGE_CURVE('',#5691,#5676,#3044,.T.);
#6994=EDGE_CURVE('',#5690,#5691,#3045,.T.);
#6995=EDGE_CURVE('',#5691,#5687,#171,.T.);
#6996=EDGE_CURVE('',#5691,#5692,#3046,.T.);
#6997=EDGE_CURVE('',#5693,#5692,#172,.T.);
#6998=EDGE_CURVE('',#5694,#5693,#173,.T.);
#6999=EDGE_CURVE('',#5694,#5688,#3047,.T.);
#7000=EDGE_CURVE('',#5695,#5690,#3048,.T.);
#7001=EDGE_CURVE('',#5692,#5695,#3049,.T.);
#7002=EDGE_CURVE('',#5696,#5685,#174,.T.);
#7003=EDGE_CURVE('',#5695,#5696,#175,.T.);
#7004=EDGE_CURVE('',#5684,#5697,#176,.T.);
#7005=EDGE_CURVE('',#5696,#5697,#177,.T.);
#7006=EDGE_CURVE('',#5698,#5693,#178,.T.);
#7007=EDGE_CURVE('',#5698,#5699,#179,.T.);
#7008=EDGE_CURVE('',#5699,#5694,#3050,.T.);
#7009=EDGE_CURVE('',#5692,#5700,#3051,.T.);
#7010=EDGE_CURVE('',#5700,#5698,#180,.T.);
#7011=EDGE_CURVE('',#5695,#5701,#3052,.T.);
#7012=EDGE_CURVE('',#5701,#5700,#3053,.T.);
#7013=EDGE_CURVE('',#5697,#5701,#181,.T.);
#7014=EDGE_CURVE('',#5682,#5702,#182,.T.);
#7015=EDGE_CURVE('',#5703,#5702,#183,.T.);
#7016=EDGE_CURVE('',#5703,#5683,#184,.T.);
#7017=EDGE_CURVE('',#5704,#5705,#185,.T.);
#7018=EDGE_CURVE('',#5706,#5705,#186,.T.);
#7019=EDGE_CURVE('',#5706,#5707,#187,.T.);
#7020=EDGE_CURVE('',#5707,#5704,#3054,.T.);
#7021=EDGE_CURVE('',#5705,#5708,#188,.T.);
#7022=EDGE_CURVE('',#5708,#5709,#3055,.T.);
#7023=EDGE_CURVE('',#5709,#5706,#189,.T.);
#7024=EDGE_CURVE('',#5708,#5710,#3056,.T.);
#7025=EDGE_CURVE('',#5710,#5711,#3057,.T.);
#7026=EDGE_CURVE('',#5711,#5709,#3058,.T.);
#7027=EDGE_CURVE('',#5702,#5711,#190,.T.);
#7028=EDGE_CURVE('',#5710,#5703,#191,.T.);
#7029=EDGE_CURVE('',#5710,#5701,#3059,.T.);
#7030=EDGE_CURVE('',#5700,#5708,#3060,.T.);
#7031=EDGE_CURVE('',#5704,#5699,#3061,.T.);
#7032=EDGE_CURVE('',#5664,#5707,#3062,.T.);
#7033=EDGE_CURVE('',#5709,#5675,#3063,.T.);
#7034=EDGE_CURVE('',#5673,#5711,#3064,.T.);
#9157=ORIENTED_EDGE('',*,*,#6955,.T.);
#9158=ORIENTED_EDGE('',*,*,#6956,.F.);
#9159=ORIENTED_EDGE('',*,*,#6957,.T.);
#9160=ORIENTED_EDGE('',*,*,#6958,.T.);
#9161=ORIENTED_EDGE('',*,*,#6959,.T.);
#9162=ORIENTED_EDGE('',*,*,#6960,.F.);
#9163=ORIENTED_EDGE('',*,*,#6961,.T.);
#9164=ORIENTED_EDGE('',*,*,#6962,.T.);
#9165=ORIENTED_EDGE('',*,*,#6960,.T.);
#9166=ORIENTED_EDGE('',*,*,#6963,.T.);
#9167=ORIENTED_EDGE('',*,*,#6964,.T.);
#9168=ORIENTED_EDGE('',*,*,#6965,.T.);
#9169=ORIENTED_EDGE('',*,*,#6966,.T.);
#9170=ORIENTED_EDGE('',*,*,#6967,.T.);
#9171=ORIENTED_EDGE('',*,*,#6964,.F.);
#9172=ORIENTED_EDGE('',*,*,#6968,.T.);
#9173=ORIENTED_EDGE('',*,*,#6956,.T.);
#9174=ORIENTED_EDGE('',*,*,#6969,.T.);
#9175=ORIENTED_EDGE('',*,*,#6966,.F.);
#9176=ORIENTED_EDGE('',*,*,#6970,.T.);
#9177=ORIENTED_EDGE('',*,*,#6957,.F.);
#9178=ORIENTED_EDGE('',*,*,#6970,.F.);
#9179=ORIENTED_EDGE('',*,*,#6971,.T.);
#9180=ORIENTED_EDGE('',*,*,#6972,.F.);
#9181=ORIENTED_EDGE('',*,*,#6973,.F.);
#9182=ORIENTED_EDGE('',*,*,#6974,.T.);
#9183=ORIENTED_EDGE('',*,*,#6968,.F.);
#9184=ORIENTED_EDGE('',*,*,#6975,.F.);
#9185=ORIENTED_EDGE('',*,*,#6976,.F.);
#9186=ORIENTED_EDGE('',*,*,#6971,.F.);
#9187=ORIENTED_EDGE('',*,*,#6963,.F.);
#9188=ORIENTED_EDGE('',*,*,#6959,.F.);
#9189=ORIENTED_EDGE('',*,*,#6977,.T.);
#9190=ORIENTED_EDGE('',*,*,#6978,.F.);
#9191=ORIENTED_EDGE('',*,*,#6979,.F.);
#9192=ORIENTED_EDGE('',*,*,#6975,.T.);
#9193=ORIENTED_EDGE('',*,*,#6962,.F.);
#9194=ORIENTED_EDGE('',*,*,#6980,.F.);
#9195=ORIENTED_EDGE('',*,*,#6981,.F.);
#9196=ORIENTED_EDGE('',*,*,#6982,.F.);
#9197=ORIENTED_EDGE('',*,*,#6983,.F.);
#9198=ORIENTED_EDGE('',*,*,#6984,.F.);
#9199=ORIENTED_EDGE('',*,*,#6985,.F.);
#9200=ORIENTED_EDGE('',*,*,#6977,.F.);
#9201=ORIENTED_EDGE('',*,*,#6973,.T.);
#9202=ORIENTED_EDGE('',*,*,#6986,.F.);
#9203=ORIENTED_EDGE('',*,*,#6987,.T.);
#9204=ORIENTED_EDGE('',*,*,#6988,.T.);
#9205=ORIENTED_EDGE('',*,*,#6989,.T.);
#9206=ORIENTED_EDGE('',*,*,#6990,.F.);
#9207=ORIENTED_EDGE('',*,*,#6978,.T.);
#9208=ORIENTED_EDGE('',*,*,#6985,.T.);
#9209=ORIENTED_EDGE('',*,*,#6990,.T.);
#9210=ORIENTED_EDGE('',*,*,#6991,.T.);
#9211=ORIENTED_EDGE('',*,*,#6992,.T.);
#9212=ORIENTED_EDGE('',*,*,#6979,.T.);
#9213=ORIENTED_EDGE('',*,*,#6993,.T.);
#9214=ORIENTED_EDGE('',*,*,#6976,.T.);
#9215=ORIENTED_EDGE('',*,*,#6992,.F.);
#9216=ORIENTED_EDGE('',*,*,#6994,.T.);
#9217=ORIENTED_EDGE('',*,*,#6986,.T.);
#9218=ORIENTED_EDGE('',*,*,#6972,.T.);
#9219=ORIENTED_EDGE('',*,*,#6993,.F.);
#9220=ORIENTED_EDGE('',*,*,#6995,.T.);
#9221=ORIENTED_EDGE('',*,*,#6987,.F.);
#9222=ORIENTED_EDGE('',*,*,#6995,.F.);
#9223=ORIENTED_EDGE('',*,*,#6996,.T.);
#9224=ORIENTED_EDGE('',*,*,#6997,.F.);
#9225=ORIENTED_EDGE('',*,*,#6998,.F.);
#9226=ORIENTED_EDGE('',*,*,#6999,.T.);
#9227=ORIENTED_EDGE('',*,*,#6994,.F.);
#9228=ORIENTED_EDGE('',*,*,#7000,.F.);
#9229=ORIENTED_EDGE('',*,*,#7001,.F.);
#9230=ORIENTED_EDGE('',*,*,#6996,.F.);
#9231=ORIENTED_EDGE('',*,*,#6991,.F.);
#9232=ORIENTED_EDGE('',*,*,#6989,.F.);
#9233=ORIENTED_EDGE('',*,*,#6984,.T.);
#9234=ORIENTED_EDGE('',*,*,#7002,.F.);
#9235=ORIENTED_EDGE('',*,*,#7003,.F.);
#9236=ORIENTED_EDGE('',*,*,#7000,.T.);
#9237=ORIENTED_EDGE('',*,*,#7004,.T.);
#9238=ORIENTED_EDGE('',*,*,#7005,.F.);
#9239=ORIENTED_EDGE('',*,*,#7002,.T.);
#9240=ORIENTED_EDGE('',*,*,#6983,.T.);
#9241=ORIENTED_EDGE('',*,*,#6998,.T.);
#9242=ORIENTED_EDGE('',*,*,#7006,.F.);
#9243=ORIENTED_EDGE('',*,*,#7007,.T.);
#9244=ORIENTED_EDGE('',*,*,#7008,.T.);
#9245=ORIENTED_EDGE('',*,*,#7006,.T.);
#9246=ORIENTED_EDGE('',*,*,#6997,.T.);
#9247=ORIENTED_EDGE('',*,*,#7009,.T.);
#9248=ORIENTED_EDGE('',*,*,#7010,.T.);
#9249=ORIENTED_EDGE('',*,*,#7009,.F.);
#9250=ORIENTED_EDGE('',*,*,#7001,.T.);
#9251=ORIENTED_EDGE('',*,*,#7011,.T.);
#9252=ORIENTED_EDGE('',*,*,#7012,.T.);
#9253=ORIENTED_EDGE('',*,*,#7005,.T.);
#9254=ORIENTED_EDGE('',*,*,#7013,.T.);
#9255=ORIENTED_EDGE('',*,*,#7011,.F.);
#9256=ORIENTED_EDGE('',*,*,#7003,.T.);
#9257=ORIENTED_EDGE('',*,*,#7014,.T.);
#9258=ORIENTED_EDGE('',*,*,#7015,.F.);
#9259=ORIENTED_EDGE('',*,*,#7016,.T.);
#9260=ORIENTED_EDGE('',*,*,#6981,.T.);
#9261=ORIENTED_EDGE('',*,*,#7017,.T.);
#9262=ORIENTED_EDGE('',*,*,#7018,.F.);
#9263=ORIENTED_EDGE('',*,*,#7019,.T.);
#9264=ORIENTED_EDGE('',*,*,#7020,.T.);
#9265=ORIENTED_EDGE('',*,*,#7018,.T.);
#9266=ORIENTED_EDGE('',*,*,#7021,.T.);
#9267=ORIENTED_EDGE('',*,*,#7022,.T.);
#9268=ORIENTED_EDGE('',*,*,#7023,.T.);
#9269=ORIENTED_EDGE('',*,*,#7022,.F.);
#9270=ORIENTED_EDGE('',*,*,#7024,.T.);
#9271=ORIENTED_EDGE('',*,*,#7025,.T.);
#9272=ORIENTED_EDGE('',*,*,#7026,.T.);
#9273=ORIENTED_EDGE('',*,*,#7015,.T.);
#9274=ORIENTED_EDGE('',*,*,#7027,.T.);
#9275=ORIENTED_EDGE('',*,*,#7025,.F.);
#9276=ORIENTED_EDGE('',*,*,#7028,.T.);
#9277=ORIENTED_EDGE('',*,*,#7004,.F.);
#9278=ORIENTED_EDGE('',*,*,#6982,.T.);
#9279=ORIENTED_EDGE('',*,*,#7016,.F.);
#9280=ORIENTED_EDGE('',*,*,#7028,.F.);
#9281=ORIENTED_EDGE('',*,*,#7029,.T.);
#9282=ORIENTED_EDGE('',*,*,#7013,.F.);
#9283=ORIENTED_EDGE('',*,*,#7012,.F.);
#9284=ORIENTED_EDGE('',*,*,#7029,.F.);
#9285=ORIENTED_EDGE('',*,*,#7024,.F.);
#9286=ORIENTED_EDGE('',*,*,#7030,.F.);
#9287=ORIENTED_EDGE('',*,*,#7010,.F.);
#9288=ORIENTED_EDGE('',*,*,#7030,.T.);
#9289=ORIENTED_EDGE('',*,*,#7021,.F.);
#9290=ORIENTED_EDGE('',*,*,#7017,.F.);
#9291=ORIENTED_EDGE('',*,*,#7031,.T.);
#9292=ORIENTED_EDGE('',*,*,#7007,.F.);
#9293=ORIENTED_EDGE('',*,*,#6955,.F.);
#9294=ORIENTED_EDGE('',*,*,#7032,.T.);
#9295=ORIENTED_EDGE('',*,*,#7019,.F.);
#9296=ORIENTED_EDGE('',*,*,#7023,.F.);
#9297=ORIENTED_EDGE('',*,*,#7033,.T.);
#9298=ORIENTED_EDGE('',*,*,#6969,.F.);
#9299=ORIENTED_EDGE('',*,*,#6958,.F.);
#9300=ORIENTED_EDGE('',*,*,#6974,.F.);
#9301=ORIENTED_EDGE('',*,*,#6988,.F.);
#9302=ORIENTED_EDGE('',*,*,#6999,.F.);
#9303=ORIENTED_EDGE('',*,*,#7008,.F.);
#9304=ORIENTED_EDGE('',*,*,#7031,.F.);
#9305=ORIENTED_EDGE('',*,*,#7020,.F.);
#9306=ORIENTED_EDGE('',*,*,#7032,.F.);
#9307=ORIENTED_EDGE('',*,*,#6965,.F.);
#9308=ORIENTED_EDGE('',*,*,#7034,.T.);
#9309=ORIENTED_EDGE('',*,*,#7027,.F.);
#9310=ORIENTED_EDGE('',*,*,#7014,.F.);
#9311=ORIENTED_EDGE('',*,*,#6980,.T.);
#9312=ORIENTED_EDGE('',*,*,#6961,.F.);
#9313=ORIENTED_EDGE('',*,*,#6967,.F.);
#9314=ORIENTED_EDGE('',*,*,#7033,.F.);
#9315=ORIENTED_EDGE('',*,*,#7026,.F.);
#9316=ORIENTED_EDGE('',*,*,#7034,.F.);
#12637=PLANE('',#14096);
#12638=PLANE('',#14098);
#12639=PLANE('',#14100);
#12640=PLANE('',#14101);
#12641=PLANE('',#14103);
#12642=PLANE('',#14105);
#12643=PLANE('',#14106);
#12644=PLANE('',#14108);
#12645=PLANE('',#14111);
#12646=PLANE('',#14113);
#13102=ADVANCED_FACE('',(#1339),#431,.T.);
#13103=ADVANCED_FACE('',(#1340),#432,.T.);
#13104=ADVANCED_FACE('',(#1341),#433,.T.);
#13105=ADVANCED_FACE('',(#1342),#12637,.T.);
#13106=ADVANCED_FACE('',(#1343),#434,.T.);
#13107=ADVANCED_FACE('',(#1344),#668,.T.);
#13108=ADVANCED_FACE('',(#1345),#12638,.T.);
#13109=ADVANCED_FACE('',(#1346),#669,.T.);
#13110=ADVANCED_FACE('',(#1347),#12639,.F.);
#13111=ADVANCED_FACE('',(#1348),#435,.T.);
#13112=ADVANCED_FACE('',(#1349),#436,.T.);
#13113=ADVANCED_FACE('',(#1350),#437,.T.);
#13114=ADVANCED_FACE('',(#1351),#12640,.T.);
#13115=ADVANCED_FACE('',(#1352),#438,.T.);
#13116=ADVANCED_FACE('',(#1353),#670,.T.);
#13117=ADVANCED_FACE('',(#1354),#12641,.T.);
#13118=ADVANCED_FACE('',(#1355),#671,.T.);
#13119=ADVANCED_FACE('',(#1356),#439,.T.);
#13120=ADVANCED_FACE('',(#1357),#440,.T.);
#13121=ADVANCED_FACE('',(#1358),#441,.T.);
#13122=ADVANCED_FACE('',(#1359),#12642,.T.);
#13123=ADVANCED_FACE('',(#1360),#442,.T.);
#13124=ADVANCED_FACE('',(#1361),#443,.T.);
#13125=ADVANCED_FACE('',(#1362),#444,.T.);
#13126=ADVANCED_FACE('',(#1363),#445,.T.);
#13127=ADVANCED_FACE('',(#1364),#12643,.T.);
#13128=ADVANCED_FACE('',(#1365),#446,.T.);
#13129=ADVANCED_FACE('',(#1366),#672,.T.);
#13130=ADVANCED_FACE('',(#1367),#12644,.T.);
#13131=ADVANCED_FACE('',(#1368),#673,.T.);
#13132=ADVANCED_FACE('',(#1369),#674,.T.);
#13133=ADVANCED_FACE('',(#1370),#12645,.T.);
#13134=ADVANCED_FACE('',(#1371),#675,.T.);
#13135=ADVANCED_FACE('',(#1372),#12646,.T.);
#13806=CLOSED_SHELL('',(#13102,#13103,#13104,#13105,#13106,#13107,#13108,
#13109,#13110,#13111,#13112,#13113,#13114,#13115,#13116,#13117,#13118,#13119,
#13120,#13121,#13122,#13123,#13124,#13125,#13126,#13127,#13128,#13129,#13130,
#13131,#13132,#13133,#13134,#13135));
#14095=AXIS2_PLACEMENT_3D('',#20630,#15377,#15378);
#14096=AXIS2_PLACEMENT_3D('',#20926,#15382,#15383);
#14097=AXIS2_PLACEMENT_3D('',#20968,#15387,#15388);
#14098=AXIS2_PLACEMENT_3D('',#21026,#15391,#15392);
#14099=AXIS2_PLACEMENT_3D('',#21030,#15395,#15396);
#14100=AXIS2_PLACEMENT_3D('',#21086,#15398,#15399);
#14101=AXIS2_PLACEMENT_3D('',#21282,#15408,#15409);
#14102=AXIS2_PLACEMENT_3D('',#21316,#15412,#15413);
#14103=AXIS2_PLACEMENT_3D('',#21374,#15416,#15417);
#14104=AXIS2_PLACEMENT_3D('',#21378,#15420,#15421);
#14105=AXIS2_PLACEMENT_3D('',#21616,#15424,#15425);
#14106=AXIS2_PLACEMENT_3D('',#21936,#15430,#15431);
#14107=AXIS2_PLACEMENT_3D('',#21978,#15435,#15436);
#14108=AXIS2_PLACEMENT_3D('',#21980,#15438,#15439);
#14109=AXIS2_PLACEMENT_3D('',#21982,#15441,#15442);
#14110=AXIS2_PLACEMENT_3D('',#21984,#15444,#15445);
#14111=AXIS2_PLACEMENT_3D('',#21987,#15448,#15449);
#14112=AXIS2_PLACEMENT_3D('',#21988,#15450,#15451);
#14113=AXIS2_PLACEMENT_3D('',#21990,#15453,#15454);
#15377=DIRECTION('axis',(0.,0.,1.));
#15378=DIRECTION('refdir',(1.,0.,0.));
#15379=DIRECTION('',(-0.707106781186481,0.,0.707106781186614));
#15380=DIRECTION('',(0.707106781186525,0.,-0.70710678118657));
#15381=DIRECTION('',(-0.707106781186548,0.,0.707106781186548));
#15382=DIRECTION('center_axis',(0.707106781186548,0.,0.707106781186548));
#15383=DIRECTION('ref_axis',(0.707106781186548,0.,-0.707106781186548));
#15384=DIRECTION('',(-0.707106781186548,0.,0.707106781186548));
#15385=DIRECTION('',(0.,-1.,0.));
#15386=DIRECTION('',(0.,1.,0.));
#15387=DIRECTION('center_axis',(0.,0.,-1.));
#15388=DIRECTION('ref_axis',(0.707106781186548,0.707106781186548,0.));
#15389=DIRECTION('',(0.,0.,-1.));
#15390=DIRECTION('',(0.,0.,1.));
#15391=DIRECTION('center_axis',(1.,0.,0.));
#15392=DIRECTION('ref_axis',(0.,0.,-1.));
#15393=DIRECTION('',(0.,0.,1.));
#15394=DIRECTION('',(0.,-1.,0.));
#15395=DIRECTION('center_axis',(0.,0.,1.));
#15396=DIRECTION('ref_axis',(0.707106781186548,-0.707106781186548,0.));
#15397=DIRECTION('',(0.,0.,-1.));
#15398=DIRECTION('center_axis',(0.,1.,0.));
#15399=DIRECTION('ref_axis',(1.,0.,0.));
#15400=DIRECTION('',(1.,0.,0.));
#15401=DIRECTION('',(0.707106781186492,0.,0.707106781186603));
#15402=DIRECTION('',(0.,0.,1.));
#15403=DIRECTION('',(-0.707106781186525,0.,0.70710678118657));
#15404=DIRECTION('',(-1.,0.,0.));
#15405=DIRECTION('',(-0.707106781186481,0.,-0.707106781186614));
#15406=DIRECTION('',(0.707106781186525,0.,0.70710678118657));
#15407=DIRECTION('',(0.70710678118661,0.,0.707106781186485));
#15408=DIRECTION('center_axis',(0.707106781186548,0.,-0.707106781186548));
#15409=DIRECTION('ref_axis',(-0.707106781186548,0.,-0.707106781186548));
#15410=DIRECTION('',(0.707106781186548,0.,0.707106781186548));
#15411=DIRECTION('',(0.,1.,0.));
#15412=DIRECTION('center_axis',(-1.,0.,0.));
#15413=DIRECTION('ref_axis',(0.,0.707106781186532,-0.707106781186563));
#15414=DIRECTION('',(-1.,0.,0.));
#15415=DIRECTION('',(1.,0.,0.));
#15416=DIRECTION('center_axis',(0.,0.,-1.));
#15417=DIRECTION('ref_axis',(-1.,0.,0.));
#15418=DIRECTION('',(1.,0.,0.));
#15419=DIRECTION('',(0.,-1.,0.));
#15420=DIRECTION('center_axis',(1.,0.,0.));
#15421=DIRECTION('ref_axis',(0.,-0.707106781186532,-0.707106781186563));
#15422=DIRECTION('',(0.707106781186525,0.,-0.70710678118657));
#15423=DIRECTION('',(-0.707106781186548,0.,0.707106781186548));
#15424=DIRECTION('center_axis',(-0.707106781186548,0.,-0.707106781186548));
#15425=DIRECTION('ref_axis',(-0.707106781186548,0.,0.707106781186548));
#15426=DIRECTION('',(-0.707106781186548,0.,0.707106781186548));
#15427=DIRECTION('',(0.,1.,0.));
#15428=DIRECTION('',(-0.707106781186492,0.,-0.707106781186603));
#15429=DIRECTION('',(0.707106781186563,0.,0.707106781186532));
#15430=DIRECTION('center_axis',(-0.707106781186548,0.,0.707106781186548));
#15431=DIRECTION('ref_axis',(0.707106781186548,0.,0.707106781186548));
#15432=DIRECTION('',(0.,-1.,0.));
#15433=DIRECTION('',(0.707106781186563,0.,0.707106781186532));
#15434=DIRECTION('',(0.,1.,0.));
#15435=DIRECTION('center_axis',(0.,0.,-1.));
#15436=DIRECTION('ref_axis',(-0.707106781186563,-0.707106781186532,0.));
#15437=DIRECTION('',(0.,0.,-1.));
#15438=DIRECTION('center_axis',(-1.,0.,0.));
#15439=DIRECTION('ref_axis',(0.,0.,1.));
#15440=DIRECTION('',(0.,0.,1.));
#15441=DIRECTION('center_axis',(0.,0.,1.));
#15442=DIRECTION('ref_axis',(-0.707106781186563,0.707106781186532,0.));
#15443=DIRECTION('',(0.,0.,-1.));
#15444=DIRECTION('center_axis',(1.,0.,0.));
#15445=DIRECTION('ref_axis',(0.,0.70710678118654,0.707106781186555));
#15446=DIRECTION('',(-1.,0.,0.));
#15447=DIRECTION('',(1.,0.,0.));
#15448=DIRECTION('center_axis',(0.,1.,0.));
#15449=DIRECTION('ref_axis',(0.,0.,1.));
#15450=DIRECTION('center_axis',(-1.,0.,0.));
#15451=DIRECTION('ref_axis',(0.,-0.70710678118654,0.707106781186555));
#15452=DIRECTION('',(-1.,0.,0.));
#15453=DIRECTION('center_axis',(0.,0.,1.));
#15454=DIRECTION('ref_axis',(1.,0.,0.));
#20630=CARTESIAN_POINT('',(0.,0.,0.));
#20631=CARTESIAN_POINT('Ctrl Pts',(176.747537170301,126.999429809249,43.6801990080023));
#20632=CARTESIAN_POINT('Ctrl Pts',(176.745869694655,126.999493365079,43.678516554556));
#20633=CARTESIAN_POINT('Ctrl Pts',(176.733667226185,126.999932122919,43.6661745561527));
#20634=CARTESIAN_POINT('Ctrl Pts',(176.720285125676,126.999995921784,43.6526083802442));
#20635=CARTESIAN_POINT('Ctrl Pts',(176.718122408304,127.,43.6504214071384));
#20636=CARTESIAN_POINT('Ctrl Pts',(176.717705939749,127.,43.65));
#20637=CARTESIAN_POINT('Ctrl Pts',(176.841757782868,126.999429809249,43.5859783954351));
#20638=CARTESIAN_POINT('Ctrl Pts',(176.840085314622,126.999493365079,43.584300934589));
#20639=CARTESIAN_POINT('Ctrl Pts',(176.827829514792,126.999932122919,43.5720122675463));
#20640=CARTESIAN_POINT('Ctrl Pts',(176.814395290254,126.999995921784,43.5584982156664));
#20641=CARTESIAN_POINT('Ctrl Pts',(176.812222074582,127.,43.5563217408604));
#20642=CARTESIAN_POINT('Ctrl Pts',(176.811803959832,127.,43.5559019799162));
#20643=CARTESIAN_POINT('Ctrl Pts',(176.935978395435,126.999429809249,43.4917577828678));
#20644=CARTESIAN_POINT('Ctrl Pts',(176.934300934589,126.999493365079,43.490085314622));
#20645=CARTESIAN_POINT('Ctrl Pts',(176.921971487686,127.000007610143,43.4778295147916));
#20646=CARTESIAN_POINT('Ctrl Pts',(176.908492562627,126.999950474695,43.4643952902542));
#20647=CARTESIAN_POINT('Ctrl Pts',(176.90632174086,127.,43.4622220745824));
#20648=CARTESIAN_POINT('Ctrl Pts',(176.905901979916,127.,43.4618039598324));
#20649=CARTESIAN_POINT('Ctrl Pts',(177.030199008002,126.999429809249,43.3975371703006));
#20650=CARTESIAN_POINT('Ctrl Pts',(177.028516554556,126.999493365079,43.395869694655));
#20651=CARTESIAN_POINT('Ctrl Pts',(177.016174556153,126.999932122919,43.3836672261852));
#20652=CARTESIAN_POINT('Ctrl Pts',(177.002608380244,126.999995921784,43.3702851256763));
#20653=CARTESIAN_POINT('Ctrl Pts',(177.000421407138,127.,43.3681224083043));
#20654=CARTESIAN_POINT('Ctrl Pts',(177.,127.,43.3677059397485));
#20655=CARTESIAN_POINT('',(176.717705939749,127.,43.65));
#20656=CARTESIAN_POINT('',(176.747537170301,126.999429809249,43.6801990080023));
#20657=CARTESIAN_POINT('Ctrl Pts',(176.717705939749,127.,43.65));
#20658=CARTESIAN_POINT('Ctrl Pts',(176.717872698805,127.,43.650168736525));
#20659=CARTESIAN_POINT('Ctrl Pts',(176.718042672762,126.999999960859,43.6503407294752));
#20660=CARTESIAN_POINT('Ctrl Pts',(176.718271119852,126.999999795533,43.6505719684178));
#20661=CARTESIAN_POINT('Ctrl Pts',(176.718523239385,126.999999613074,43.6508271691041));
#20662=CARTESIAN_POINT('Ctrl Pts',(176.718846507485,126.99999928102,43.6511544591101));
#20663=CARTESIAN_POINT('Ctrl Pts',(176.719268262893,126.999998436683,43.6515815512717));
#20664=CARTESIAN_POINT('Ctrl Pts',(176.719739279202,126.999997493728,43.6520585276647));
#20665=CARTESIAN_POINT('Ctrl Pts',(176.720332661821,126.999995895344,43.6526595049513));
#20666=CARTESIAN_POINT('Ctrl Pts',(176.721034596213,126.999992899769,43.6533705073352));
#20667=CARTESIAN_POINT('Ctrl Pts',(176.721922356591,126.999989111163,43.654269736312));
#20668=CARTESIAN_POINT('Ctrl Pts',(176.72298234306,126.999982983391,43.6553435322326));
#20669=CARTESIAN_POINT('Ctrl Pts',(176.724119373636,126.999973630094,43.6564954718405));
#20670=CARTESIAN_POINT('Ctrl Pts',(176.725267024347,126.999964189434,43.6576581708371));
#20671=CARTESIAN_POINT('Ctrl Pts',(176.726487764087,126.999951463521,43.6588950097938));
#20672=CARTESIAN_POINT('Ctrl Pts',(176.727682323414,126.999936173481,43.6601053627628));
#20673=CARTESIAN_POINT('Ctrl Pts',(176.728576869224,126.999924723534,43.6610117356424));
#20674=CARTESIAN_POINT('Ctrl Pts',(176.729456205746,126.999911911841,43.6619027203553));
#20675=CARTESIAN_POINT('Ctrl Pts',(176.730305951649,126.999898173663,43.6627636895374));
#20676=CARTESIAN_POINT('Ctrl Pts',(176.731077458531,126.999885700406,43.6635453863343));
#20677=CARTESIAN_POINT('Ctrl Pts',(176.731824182401,126.999872502733,43.6643019452847));
#20678=CARTESIAN_POINT('Ctrl Pts',(176.732566882097,126.999858342121,43.665054319646));
#20679=CARTESIAN_POINT('Ctrl Pts',(176.733343831679,126.999843528486,43.6658413900453));
#20680=CARTESIAN_POINT('Ctrl Pts',(176.734123555715,126.99982752742,43.6666311424732));
#20681=CARTESIAN_POINT('Ctrl Pts',(176.734930805536,126.999809694323,43.6674485777798));
#20682=CARTESIAN_POINT('Ctrl Pts',(176.735832024149,126.999789785346,43.6683611675309));
#20683=CARTESIAN_POINT('Ctrl Pts',(176.736766994247,126.999767552882,43.6693076969592));
#20684=CARTESIAN_POINT('Ctrl Pts',(176.737717360141,126.999743173977,43.670269575142));
#20685=CARTESIAN_POINT('Ctrl Pts',(176.738959763474,126.999711303693,43.6715270283689));
#20686=CARTESIAN_POINT('Ctrl Pts',(176.740226781866,126.999675666215,43.6728089911326));
#20687=CARTESIAN_POINT('Ctrl Pts',(176.741404811927,126.999639900927,43.6740006009478));
#20688=CARTESIAN_POINT('Ctrl Pts',(176.742367569254,126.999610671373,43.6749744564707));
#20689=CARTESIAN_POINT('Ctrl Pts',(176.743267661294,126.999581516184,43.6758847018519));
#20690=CARTESIAN_POINT('Ctrl Pts',(176.744045268374,126.999555290462,43.6766709110228));
#20691=CARTESIAN_POINT('Ctrl Pts',(176.744722380664,126.999532454046,43.6773555137054));
#20692=CARTESIAN_POINT('Ctrl Pts',(176.745305724149,126.999511912239,43.6779451634335));
#20693=CARTESIAN_POINT('Ctrl Pts',(176.745779966788,126.999494873465,43.6784244138591));
#20694=CARTESIAN_POINT('Ctrl Pts',(176.746218303809,126.999479124722,43.6788673795207));
#20695=CARTESIAN_POINT('Ctrl Pts',(176.746562942419,126.999466401456,43.6792155329358));
#20696=CARTESIAN_POINT('Ctrl Pts',(176.746832907361,126.999456345864,43.6794881511433));
#20697=CARTESIAN_POINT('Ctrl Pts',(176.747083726891,126.999447003396,43.6797414357741));
#20698=CARTESIAN_POINT('Ctrl Pts',(176.74726987331,126.999439970325,43.6799293013882));
#20699=CARTESIAN_POINT('Ctrl Pts',(176.747439207675,126.999433537031,43.6801001639586));
#20700=CARTESIAN_POINT('Ctrl Pts',(176.747472215255,126.999432283018,43.6801334694242));
#20701=CARTESIAN_POINT('Ctrl Pts',(176.747504695246,126.999431047036,43.6801662412462));
#20702=CARTESIAN_POINT('Ctrl Pts',(176.747537170301,126.999429809249,43.6801990080023));
#20703=CARTESIAN_POINT('',(177.030199008002,126.999429809249,43.3975371703006));
#20704=CARTESIAN_POINT('Ctrl Pts',(177.030199008002,126.999429809249,43.3975371703006));
#20705=CARTESIAN_POINT('Ctrl Pts',(176.935978395435,126.999429809249,43.4917577828678));
#20706=CARTESIAN_POINT('Ctrl Pts',(176.841757782868,126.999429809249,43.5859783954351));
#20707=CARTESIAN_POINT('Ctrl Pts',(176.747537170301,126.999429809249,43.6801990080023));
#20708=CARTESIAN_POINT('',(177.,127.,43.3677059397485));
#20709=CARTESIAN_POINT('Ctrl Pts',(177.030199008002,126.999429809249,43.3975371703006));
#20710=CARTESIAN_POINT('Ctrl Pts',(177.030030585505,126.999436171524,43.3973702471606));
#20711=CARTESIAN_POINT('Ctrl Pts',(177.029858909386,126.999442617638,43.3972001071489));
#20712=CARTESIAN_POINT('Ctrl Pts',(177.029628057339,126.99945117313,43.396971463311));
#20713=CARTESIAN_POINT('Ctrl Pts',(177.029373282892,126.999460615197,43.3967191259022));
#20714=CARTESIAN_POINT('Ctrl Pts',(177.029046504163,126.999472627869,43.3963956021262));
#20715=CARTESIAN_POINT('Ctrl Pts',(177.028620026165,126.999487894907,43.395973543409));
#20716=CARTESIAN_POINT('Ctrl Pts',(177.0281437326,126.999504945239,43.3955021853265));
#20717=CARTESIAN_POINT('Ctrl Pts',(177.027543563761,126.999526020176,43.3949084001559));
#20718=CARTESIAN_POINT('Ctrl Pts',(177.026833440411,126.999549852402,43.394206022241));
#20719=CARTESIAN_POINT('Ctrl Pts',(177.025935290825,126.999579994917,43.3933176689235));
#20720=CARTESIAN_POINT('Ctrl Pts',(177.0248626695,126.999614390365,43.3922570121512));
#20721=CARTESIAN_POINT('Ctrl Pts',(177.023711822739,126.999648516201,43.3911193310076));
#20722=CARTESIAN_POINT('Ctrl Pts',(177.02255032393,126.9996829579,43.3899711196752));
#20723=CARTESIAN_POINT('Ctrl Pts',(177.021314608223,126.999716919438,43.3887498553891));
#20724=CARTESIAN_POINT('Ctrl Pts',(177.02010513109,126.999747324912,43.3875548864531));
#20725=CARTESIAN_POINT('Ctrl Pts',(177.019199401769,126.999770094362,43.3866600217438));
#20726=CARTESIAN_POINT('Ctrl Pts',(177.018308923963,126.999790925398,43.3857804315058));
#20727=CARTESIAN_POINT('Ctrl Pts',(177.017448288609,126.999809700632,43.384930519969));
#20728=CARTESIAN_POINT('Ctrl Pts',(177.016666887984,126.999826747316,43.3841588558682));
#20729=CARTESIAN_POINT('Ctrl Pts',(177.015910483889,126.999842123653,43.3834120480744));
#20730=CARTESIAN_POINT('Ctrl Pts',(177.015158111381,126.999856381896,43.3826693398961));
#20731=CARTESIAN_POINT('Ctrl Pts',(177.014371053415,126.999871297464,43.3818923917999));
#20732=CARTESIAN_POINT('Ctrl Pts',(177.013581145567,126.999885130105,43.3811127516123));
#20733=CARTESIAN_POINT('Ctrl Pts',(177.012763400092,126.999898178282,43.3803056659763));
#20734=CARTESIAN_POINT('Ctrl Pts',(177.011850452589,126.999912745528,43.3794046193326));
#20735=CARTESIAN_POINT('Ctrl Pts',(177.010903370168,126.999926273619,43.3784699201045));
#20736=CARTESIAN_POINT('Ctrl Pts',(177.00994078853,126.999938235568,43.3775198964634));
#20737=CARTESIAN_POINT('Ctrl Pts',(177.008682347624,126.999953874144,43.3762778733826));
#20738=CARTESIAN_POINT('Ctrl Pts',(177.007399134253,126.999966671765,43.375011353504));
#20739=CARTESIAN_POINT('Ctrl Pts',(177.006206223417,126.999975926382,43.3738338670282));
#20740=CARTESIAN_POINT('Ctrl Pts',(177.00523142736,126.999983488862,43.3728716751026));
#20741=CARTESIAN_POINT('Ctrl Pts',(177.004320197324,126.999988722094,43.3719721616102));
#20742=CARTESIAN_POINT('Ctrl Pts',(177.003533069758,126.999992198348,43.3711950841717));
#20743=CARTESIAN_POINT('Ctrl Pts',(177.002847649353,126.999995225425,43.3705184152863));
#20744=CARTESIAN_POINT('Ctrl Pts',(177.002257239447,126.999996959481,43.3699354824491));
#20745=CARTESIAN_POINT('Ctrl Pts',(177.001777334972,126.999998025673,43.369461595752));
#20746=CARTESIAN_POINT('Ctrl Pts',(177.00133376131,126.999999011149,43.3690235842967));
#20747=CARTESIAN_POINT('Ctrl Pts',(177.000985093106,126.999999440092,43.3686792256923));
#20748=CARTESIAN_POINT('Ctrl Pts',(177.000712044094,126.999999683121,43.368409497874));
#20749=CARTESIAN_POINT('Ctrl Pts',(177.000458357712,126.999999908916,43.3681588971718));
#20750=CARTESIAN_POINT('Ctrl Pts',(177.000270163794,126.999999972695,43.3679729332256));
#20751=CARTESIAN_POINT('Ctrl Pts',(177.000098987777,126.999999993876,43.3678037667735));
#20752=CARTESIAN_POINT('Ctrl Pts',(177.000065634447,126.999999998003,43.3677708050029));
#20753=CARTESIAN_POINT('Ctrl Pts',(177.000032814729,127.,43.3677383699128));
#20754=CARTESIAN_POINT('Ctrl Pts',(177.,127.,43.3677059397485));
#20755=CARTESIAN_POINT('',(176.858852969874,127.,43.5088529698743));
#20756=CARTESIAN_POINT('Ctrl Pts',(177.030199008002,122.238070190751,43.3975371703006));
#20757=CARTESIAN_POINT('Ctrl Pts',(177.028516554556,122.238006634921,43.395869694655));
#20758=CARTESIAN_POINT('Ctrl Pts',(177.016174465217,122.237567875321,43.3836671357425));
#20759=CARTESIAN_POINT('Ctrl Pts',(177.002608356514,122.237504077912,43.3702851021113));
#20760=CARTESIAN_POINT('Ctrl Pts',(177.000421407138,122.2375,43.3681224083044));
#20761=CARTESIAN_POINT('Ctrl Pts',(177.,122.2375,43.3677059397486));
#20762=CARTESIAN_POINT('Ctrl Pts',(176.935978395435,122.238070190751,43.4917577828679));
#20763=CARTESIAN_POINT('Ctrl Pts',(176.934300934589,122.238006634921,43.490085314622));
#20764=CARTESIAN_POINT('Ctrl Pts',(176.92201217661,122.237567875321,43.4778294243489));
#20765=CARTESIAN_POINT('Ctrl Pts',(176.908498191936,122.237504077912,43.4643952666892));
#20766=CARTESIAN_POINT('Ctrl Pts',(176.90632174086,122.2375,43.4622220745824));
#20767=CARTESIAN_POINT('Ctrl Pts',(176.905901979916,122.2375,43.4618039598324));
#20768=CARTESIAN_POINT('Ctrl Pts',(176.841757782868,122.238070190751,43.5859783954351));
#20769=CARTESIAN_POINT('Ctrl Pts',(176.840085314622,122.238006634921,43.5843009345891));
#20770=CARTESIAN_POINT('Ctrl Pts',(176.827829424349,122.237492398776,43.571971396334));
#20771=CARTESIAN_POINT('Ctrl Pts',(176.814395266689,122.237549527789,43.5584925388249));
#20772=CARTESIAN_POINT('Ctrl Pts',(176.812222074582,122.2375,43.5563217408604));
#20773=CARTESIAN_POINT('Ctrl Pts',(176.811803959832,122.2375,43.5559019799162));
#20774=CARTESIAN_POINT('Ctrl Pts',(176.747537170301,122.238070190751,43.6801990080024));
#20775=CARTESIAN_POINT('Ctrl Pts',(176.745869694655,122.238006634921,43.6785165545561));
#20776=CARTESIAN_POINT('Ctrl Pts',(176.733667135743,122.237567875321,43.6661744652167));
#20777=CARTESIAN_POINT('Ctrl Pts',(176.720285102111,122.237504077912,43.6526083565139));
#20778=CARTESIAN_POINT('Ctrl Pts',(176.718122408304,122.2375,43.6504214071384));
#20779=CARTESIAN_POINT('Ctrl Pts',(176.717705939749,122.2375,43.65));
#20780=CARTESIAN_POINT('',(177.,122.2375,43.3677059397486));
#20781=CARTESIAN_POINT('',(177.030199008002,122.238070190751,43.3975371703006));
#20782=CARTESIAN_POINT('Ctrl Pts',(177.,122.2375,43.3677059397486));
#20783=CARTESIAN_POINT('Ctrl Pts',(177.000168736525,122.2375,43.3678726988053));
#20784=CARTESIAN_POINT('Ctrl Pts',(177.000340729475,122.237500039141,43.3680426727623));
#20785=CARTESIAN_POINT('Ctrl Pts',(177.000571968418,122.237500204467,43.3682711198523));
#20786=CARTESIAN_POINT('Ctrl Pts',(177.000827169104,122.237500386926,43.3685232393849));
#20787=CARTESIAN_POINT('Ctrl Pts',(177.00115445911,122.23750071898,43.3688465074852));
#20788=CARTESIAN_POINT('Ctrl Pts',(177.001581551272,122.237501563317,43.3692682628933));
#20789=CARTESIAN_POINT('Ctrl Pts',(177.002058527665,122.237502506272,43.3697392792016));
#20790=CARTESIAN_POINT('Ctrl Pts',(177.002659504951,122.237504104656,43.3703326618207));
#20791=CARTESIAN_POINT('Ctrl Pts',(177.003370507335,122.237507100231,43.3710345962129));
#20792=CARTESIAN_POINT('Ctrl Pts',(177.004269736312,122.237510888837,43.3719223565912));
#20793=CARTESIAN_POINT('Ctrl Pts',(177.005343532233,122.237517016609,43.3729823430604));
#20794=CARTESIAN_POINT('Ctrl Pts',(177.006495471841,122.237526369906,43.3741193736364));
#20795=CARTESIAN_POINT('Ctrl Pts',(177.007658170837,122.237535810566,43.3752670243474));
#20796=CARTESIAN_POINT('Ctrl Pts',(177.008895009794,122.237548536479,43.3764877640871));
#20797=CARTESIAN_POINT('Ctrl Pts',(177.010105362763,122.237563826519,43.3776823234142));
#20798=CARTESIAN_POINT('Ctrl Pts',(177.011011735643,122.237575276466,43.3785768692244));
#20799=CARTESIAN_POINT('Ctrl Pts',(177.011902720356,122.237588088159,43.3794562057466));
#20800=CARTESIAN_POINT('Ctrl Pts',(177.012763689538,122.237601826337,43.3803059516489));
#20801=CARTESIAN_POINT('Ctrl Pts',(177.013545386334,122.237614299594,43.3810774585317));
#20802=CARTESIAN_POINT('Ctrl Pts',(177.014301945285,122.237627497267,43.3818241824014));
#20803=CARTESIAN_POINT('Ctrl Pts',(177.015054319646,122.237641657879,43.3825668820968));
#20804=CARTESIAN_POINT('Ctrl Pts',(177.015841390045,122.237656471514,43.3833438316793));
#20805=CARTESIAN_POINT('Ctrl Pts',(177.016631142473,122.23767247258,43.3841235557154));
#20806=CARTESIAN_POINT('Ctrl Pts',(177.01744857778,122.237690305677,43.3849308055361));
#20807=CARTESIAN_POINT('Ctrl Pts',(177.018361167531,122.237710214654,43.3858320241488));
#20808=CARTESIAN_POINT('Ctrl Pts',(177.019307696959,122.237732447118,43.3867669942467));
#20809=CARTESIAN_POINT('Ctrl Pts',(177.020269575142,122.237756826022,43.3877173601411));
#20810=CARTESIAN_POINT('Ctrl Pts',(177.021527028369,122.237788696307,43.3889597634745));
#20811=CARTESIAN_POINT('Ctrl Pts',(177.022808991133,122.237824333785,43.390226781866));
#20812=CARTESIAN_POINT('Ctrl Pts',(177.024000600948,122.237860099073,43.3914048119272));
#20813=CARTESIAN_POINT('Ctrl Pts',(177.024974456471,122.237889328627,43.3923675692547));
#20814=CARTESIAN_POINT('Ctrl Pts',(177.025884701852,122.237918483816,43.3932676612944));
#20815=CARTESIAN_POINT('Ctrl Pts',(177.026670911023,122.237944709538,43.394045268374));
#20816=CARTESIAN_POINT('Ctrl Pts',(177.027355513706,122.237967545954,43.3947223806646));
#20817=CARTESIAN_POINT('Ctrl Pts',(177.027945163434,122.237988087761,43.3953057241498));
#20818=CARTESIAN_POINT('Ctrl Pts',(177.028424413859,122.238005126535,43.395779966788));
#20819=CARTESIAN_POINT('Ctrl Pts',(177.028867379521,122.238020875278,43.3962183038092));
#20820=CARTESIAN_POINT('Ctrl Pts',(177.029215532936,122.238033598544,43.3965629424196));
#20821=CARTESIAN_POINT('Ctrl Pts',(177.029488151143,122.238043654136,43.3968329073614));
#20822=CARTESIAN_POINT('Ctrl Pts',(177.029741435774,122.238052996604,43.3970837268911));
#20823=CARTESIAN_POINT('Ctrl Pts',(177.029929301388,122.238060029675,43.3972698733102));
#20824=CARTESIAN_POINT('Ctrl Pts',(177.030100163959,122.238066462969,43.3974392076751));
#20825=CARTESIAN_POINT('Ctrl Pts',(177.030133469424,122.238067716982,43.3974722152546));
#20826=CARTESIAN_POINT('Ctrl Pts',(177.030166241246,122.238068952964,43.3975046952459));
#20827=CARTESIAN_POINT('Ctrl Pts',(177.030199008002,122.238070190751,43.3975371703006));
#20828=CARTESIAN_POINT('',(176.747537170301,122.238070190751,43.6801990080024));
#20829=CARTESIAN_POINT('Ctrl Pts',(176.747537170301,122.238070190751,43.6801990080024));
#20830=CARTESIAN_POINT('Ctrl Pts',(176.841757782868,122.238070190751,43.5859783954351));
#20831=CARTESIAN_POINT('Ctrl Pts',(176.935978395435,122.238070190751,43.4917577828679));
#20832=CARTESIAN_POINT('Ctrl Pts',(177.030199008002,122.238070190751,43.3975371703006));
#20833=CARTESIAN_POINT('',(176.717705939749,122.2375,43.65));
#20834=CARTESIAN_POINT('Ctrl Pts',(176.747537170301,122.238070190751,43.6801990080024));
#20835=CARTESIAN_POINT('Ctrl Pts',(176.747370247161,122.238063828476,43.6800305855052));
#20836=CARTESIAN_POINT('Ctrl Pts',(176.747200107149,122.238057382362,43.6798589093858));
#20837=CARTESIAN_POINT('Ctrl Pts',(176.746971463311,122.23804882687,43.6796280573389));
#20838=CARTESIAN_POINT('Ctrl Pts',(176.746719125902,122.238039384803,43.679373282892));
#20839=CARTESIAN_POINT('Ctrl Pts',(176.746395602126,122.238027372131,43.6790465041629));
#20840=CARTESIAN_POINT('Ctrl Pts',(176.745973543409,122.238012105093,43.6786200261655));
#20841=CARTESIAN_POINT('Ctrl Pts',(176.745502185327,122.237995054761,43.6781437326003));
#20842=CARTESIAN_POINT('Ctrl Pts',(176.744908400156,122.237973979824,43.6775435637607));
#20843=CARTESIAN_POINT('Ctrl Pts',(176.744206022241,122.237950147598,43.6768334404111));
#20844=CARTESIAN_POINT('Ctrl Pts',(176.743317668924,122.237920005083,43.6759352908253));
#20845=CARTESIAN_POINT('Ctrl Pts',(176.742257012151,122.237885609635,43.6748626694999));
#20846=CARTESIAN_POINT('Ctrl Pts',(176.741119331008,122.237851483799,43.6737118227386));
#20847=CARTESIAN_POINT('Ctrl Pts',(176.739971119675,122.2378170421,43.6725503239298));
#20848=CARTESIAN_POINT('Ctrl Pts',(176.738749855389,122.237783080562,43.6713146082227));
#20849=CARTESIAN_POINT('Ctrl Pts',(176.737554886453,122.237752675088,43.67010513109));
#20850=CARTESIAN_POINT('Ctrl Pts',(176.736660021744,122.237729905638,43.6691994017693));
#20851=CARTESIAN_POINT('Ctrl Pts',(176.735780431506,122.237709074602,43.6683089239629));
#20852=CARTESIAN_POINT('Ctrl Pts',(176.734930519969,122.237690299368,43.6674482886094));
#20853=CARTESIAN_POINT('Ctrl Pts',(176.734158855873,122.237673252684,43.6666668879893));
#20854=CARTESIAN_POINT('Ctrl Pts',(176.733412048084,122.237657876347,43.6659104838988));
#20855=CARTESIAN_POINT('Ctrl Pts',(176.73266933991,122.237643618104,43.665158111395));
#20856=CARTESIAN_POINT('Ctrl Pts',(176.731892391814,122.237628702536,43.6643710534291));
#20857=CARTESIAN_POINT('Ctrl Pts',(176.731112751627,122.237614869895,43.6635811455825));
#20858=CARTESIAN_POINT('Ctrl Pts',(176.730305665992,122.237601821719,43.6627634001078));
#20859=CARTESIAN_POINT('Ctrl Pts',(176.729404619349,122.237587254472,43.6618504526061));
#20860=CARTESIAN_POINT('Ctrl Pts',(176.728469920122,122.237573726382,43.6609033701865));
#20861=CARTESIAN_POINT('Ctrl Pts',(176.727519896482,122.237561764432,43.6599407885492));
#20862=CARTESIAN_POINT('Ctrl Pts',(176.726277873407,122.237546125856,43.6586823476483));
#20863=CARTESIAN_POINT('Ctrl Pts',(176.725011353533,122.237533328236,43.6573991342823));
#20864=CARTESIAN_POINT('Ctrl Pts',(176.723833867061,122.237524073618,43.6562062234503));
#20865=CARTESIAN_POINT('Ctrl Pts',(176.722871675132,122.237516511138,43.6552314273898));
#20866=CARTESIAN_POINT('Ctrl Pts',(176.721972161636,122.237511277906,43.6543201973493));
#20867=CARTESIAN_POINT('Ctrl Pts',(176.721195084193,122.237507801652,43.6535330697796));
#20868=CARTESIAN_POINT('Ctrl Pts',(176.720518415305,122.237504774575,43.6528476493719));
#20869=CARTESIAN_POINT('Ctrl Pts',(176.719935482465,122.237503040519,43.6522572394634));
#20870=CARTESIAN_POINT('Ctrl Pts',(176.719461595766,122.237501974327,43.6517773349856));
#20871=CARTESIAN_POINT('Ctrl Pts',(176.719023584308,122.237500988851,43.6513337613213));
#20872=CARTESIAN_POINT('Ctrl Pts',(176.718679225702,122.237500559908,43.6509850931152));
#20873=CARTESIAN_POINT('Ctrl Pts',(176.718409497882,122.237500316879,43.6507120441015));
#20874=CARTESIAN_POINT('Ctrl Pts',(176.718158897178,122.237500091084,43.6504583577189));
#20875=CARTESIAN_POINT('Ctrl Pts',(176.717972933231,122.237500027304,43.6502701637992));
#20876=CARTESIAN_POINT('Ctrl Pts',(176.717803766779,122.237500006124,43.6500989877827));
#20877=CARTESIAN_POINT('Ctrl Pts',(176.717770805006,122.237500001997,43.6500656344504));
#20878=CARTESIAN_POINT('Ctrl Pts',(176.717738369915,122.2375,43.6500328147306));
#20879=CARTESIAN_POINT('Ctrl Pts',(176.717705939749,122.2375,43.65));
#20880=CARTESIAN_POINT('',(176.858852969874,122.2375,43.5088529698743));
#20881=CARTESIAN_POINT('Ctrl Pts',(176.747537170301,122.238070190751,43.6801990080024));
#20882=CARTESIAN_POINT('Ctrl Pts',(176.878145139865,122.243048313183,43.8119801402103));
#20883=CARTESIAN_POINT('Ctrl Pts',(177.142745845888,122.319065602083,44.0669582028244));
#20884=CARTESIAN_POINT('Ctrl Pts',(177.429161451671,122.559475348238,44.3164670343898));
#20885=CARTESIAN_POINT('Ctrl Pts',(177.574122249711,122.816490807511,44.43105315404));
#20886=CARTESIAN_POINT('Ctrl Pts',(177.6,122.964234224196,44.45));
#20887=CARTESIAN_POINT('Ctrl Pts',(177.6,123.0375,44.45));
#20888=CARTESIAN_POINT('Ctrl Pts',(176.841757782868,122.238070190751,43.5859783954351));
#20889=CARTESIAN_POINT('Ctrl Pts',(176.972756806647,122.243048313183,43.7173684734285));
#20890=CARTESIAN_POINT('Ctrl Pts',(177.234149964867,122.319065602083,43.9755540838455));
#20891=CARTESIAN_POINT('Ctrl Pts',(177.508263312577,122.559475348238,44.2373651734836));
#20892=CARTESIAN_POINT('Ctrl Pts',(177.643099217821,122.816490807511,44.3620761859304));
#20893=CARTESIAN_POINT('Ctrl Pts',(177.666666666667,122.964234224196,44.3833333333333));
#20894=CARTESIAN_POINT('Ctrl Pts',(177.666666666667,123.0375,44.3833333333333));
#20895=CARTESIAN_POINT('Ctrl Pts',(176.935978395435,122.238070190751,43.4917577828679));
#20896=CARTESIAN_POINT('Ctrl Pts',(177.067368473429,122.243048313183,43.6227568066467));
#20897=CARTESIAN_POINT('Ctrl Pts',(177.325554083845,122.319065602083,43.8841499648667));
#20898=CARTESIAN_POINT('Ctrl Pts',(177.587365173484,122.559475348238,44.1582633125774));
#20899=CARTESIAN_POINT('Ctrl Pts',(177.71207618593,122.816490807511,44.2930992178208));
#20900=CARTESIAN_POINT('Ctrl Pts',(177.733333333333,122.964234224196,44.3166666666667));
#20901=CARTESIAN_POINT('Ctrl Pts',(177.733333333333,123.0375,44.3166666666667));
#20902=CARTESIAN_POINT('Ctrl Pts',(177.030199008002,122.238070190751,43.3975371703006));
#20903=CARTESIAN_POINT('Ctrl Pts',(177.16198014021,122.243048313183,43.5281451398648));
#20904=CARTESIAN_POINT('Ctrl Pts',(177.416958202824,122.319065602083,43.7927458458878));
#20905=CARTESIAN_POINT('Ctrl Pts',(177.66646703439,122.559475348238,44.0791614516713));
#20906=CARTESIAN_POINT('Ctrl Pts',(177.78105315404,122.816490807511,44.2241222497112));
#20907=CARTESIAN_POINT('Ctrl Pts',(177.8,122.964234224196,44.25));
#20908=CARTESIAN_POINT('Ctrl Pts',(177.8,123.0375,44.25));
#20909=CARTESIAN_POINT('',(177.8,123.0375,44.25));
#20910=CARTESIAN_POINT('Ctrl Pts',(177.030199008002,122.238070190751,43.3975371703006));
#20911=CARTESIAN_POINT('Ctrl Pts',(177.16198014021,122.243048313183,43.5281451398648));
#20912=CARTESIAN_POINT('Ctrl Pts',(177.416958202824,122.319065602083,43.7927458458878));
#20913=CARTESIAN_POINT('Ctrl Pts',(177.66646703439,122.559475348238,44.0791614516713));
#20914=CARTESIAN_POINT('Ctrl Pts',(177.78105315404,122.816490807511,44.2241222497112));
#20915=CARTESIAN_POINT('Ctrl Pts',(177.8,122.964234224196,44.25));
#20916=CARTESIAN_POINT('Ctrl Pts',(177.8,123.0375,44.25));
#20917=CARTESIAN_POINT('',(177.6,123.0375,44.45));
#20918=CARTESIAN_POINT('',(177.8,123.0375,44.25));
#20919=CARTESIAN_POINT('Ctrl Pts',(177.6,123.0375,44.45));
#20920=CARTESIAN_POINT('Ctrl Pts',(177.6,122.964234224196,44.45));
#20921=CARTESIAN_POINT('Ctrl Pts',(177.574122249711,122.816490807511,44.43105315404));
#20922=CARTESIAN_POINT('Ctrl Pts',(177.429161451671,122.559475348238,44.3164670343898));
#20923=CARTESIAN_POINT('Ctrl Pts',(177.142745845888,122.319065602083,44.0669582028244));
#20924=CARTESIAN_POINT('Ctrl Pts',(176.878145139865,122.243048313183,43.8119801402103));
#20925=CARTESIAN_POINT('Ctrl Pts',(176.747537170301,122.238070190751,43.6801990080024));
#20926=CARTESIAN_POINT('Origin',(177.7,122.2375,44.35));
#20927=CARTESIAN_POINT('',(177.8,126.2,44.25));
#20928=CARTESIAN_POINT('',(177.6,126.2,44.45));
#20929=CARTESIAN_POINT('',(177.8,126.2,44.25));
#20930=CARTESIAN_POINT('',(177.6,122.2375,44.45));
#20931=CARTESIAN_POINT('',(177.8,122.2375,44.25));
#20932=CARTESIAN_POINT('Ctrl Pts',(177.030199008002,126.999429809249,43.3975371703006));
#20933=CARTESIAN_POINT('Ctrl Pts',(177.227870706314,126.991962625601,43.5934491246469));
#20934=CARTESIAN_POINT('Ctrl Pts',(177.539136404472,126.85217227369,43.9258693224329));
#20935=CARTESIAN_POINT('Ctrl Pts',(177.766798305442,126.497803729337,44.2039283446181));
#20936=CARTESIAN_POINT('Ctrl Pts',(177.8,126.297687701072,44.25));
#20937=CARTESIAN_POINT('Ctrl Pts',(177.8,126.2,44.25));
#20938=CARTESIAN_POINT('Ctrl Pts',(176.935978395435,126.999429809249,43.4917577828678));
#20939=CARTESIAN_POINT('Ctrl Pts',(177.133063512425,126.991962625601,43.688256318536));
#20940=CARTESIAN_POINT('Ctrl Pts',(177.451380710459,126.85217227369,44.0136250164458));
#20941=CARTESIAN_POINT('Ctrl Pts',(177.695841651834,126.497803729337,44.274884998226));
#20942=CARTESIAN_POINT('Ctrl Pts',(177.733333333333,126.297687701072,44.3166666666667));
#20943=CARTESIAN_POINT('Ctrl Pts',(177.733333333333,126.2,44.3166666666667));
#20944=CARTESIAN_POINT('Ctrl Pts',(176.841757782868,126.999429809249,43.5859783954351));
#20945=CARTESIAN_POINT('Ctrl Pts',(177.038256318536,126.991962625601,43.7830635124252));
#20946=CARTESIAN_POINT('Ctrl Pts',(177.363625016446,126.85217227369,44.1013807104587));
#20947=CARTESIAN_POINT('Ctrl Pts',(177.624884998226,126.497803729337,44.3458416518339));
#20948=CARTESIAN_POINT('Ctrl Pts',(177.666666666667,126.297687701072,44.3833333333333));
#20949=CARTESIAN_POINT('Ctrl Pts',(177.666666666667,126.2,44.3833333333333));
#20950=CARTESIAN_POINT('Ctrl Pts',(176.747537170301,126.999429809249,43.6801990080023));
#20951=CARTESIAN_POINT('Ctrl Pts',(176.943449124647,126.991962625601,43.8778707063143));
#20952=CARTESIAN_POINT('Ctrl Pts',(177.275869322433,126.85217227369,44.1891364044717));
#20953=CARTESIAN_POINT('Ctrl Pts',(177.553928344618,126.497803729337,44.4167983054418));
#20954=CARTESIAN_POINT('Ctrl Pts',(177.6,126.297687701072,44.45));
#20955=CARTESIAN_POINT('Ctrl Pts',(177.6,126.2,44.45));
#20956=CARTESIAN_POINT('Ctrl Pts',(176.747537170301,126.999429809249,43.6801990080023));
#20957=CARTESIAN_POINT('Ctrl Pts',(176.943449124647,126.991962625601,43.8778707063143));
#20958=CARTESIAN_POINT('Ctrl Pts',(177.275869322433,126.85217227369,44.1891364044717));
#20959=CARTESIAN_POINT('Ctrl Pts',(177.553928344618,126.497803729337,44.4167983054418));
#20960=CARTESIAN_POINT('Ctrl Pts',(177.6,126.297687701072,44.45));
#20961=CARTESIAN_POINT('Ctrl Pts',(177.6,126.2,44.45));
#20962=CARTESIAN_POINT('Ctrl Pts',(177.8,126.2,44.25));
#20963=CARTESIAN_POINT('Ctrl Pts',(177.8,126.297687701072,44.25));
#20964=CARTESIAN_POINT('Ctrl Pts',(177.766798305442,126.497803729337,44.2039283446181));
#20965=CARTESIAN_POINT('Ctrl Pts',(177.539136404472,126.85217227369,43.9258693224329));
#20966=CARTESIAN_POINT('Ctrl Pts',(177.227870706314,126.991962625601,43.5934491246469));
#20967=CARTESIAN_POINT('Ctrl Pts',(177.030199008002,126.999429809249,43.3975371703006));
#20968=CARTESIAN_POINT('Origin',(177.,126.2,6.35000000000001));
#20969=CARTESIAN_POINT('',(177.8,126.2,-107.75));
#20970=CARTESIAN_POINT('',(177.8,126.2,6.35000000000001));
#20971=CARTESIAN_POINT('',(177.030199008002,126.999429809249,-106.897537170301));
#20972=CARTESIAN_POINT('Ctrl Pts',(177.030199008002,126.999429809249,-106.897537170301));
#20973=CARTESIAN_POINT('Ctrl Pts',(177.227870706314,126.991962625601,-107.093449124647));
#20974=CARTESIAN_POINT('Ctrl Pts',(177.539138426476,126.852173302019,-107.425873068733));
#20975=CARTESIAN_POINT('Ctrl Pts',(177.766802032304,126.49780856488,-107.703932070819));
#20976=CARTESIAN_POINT('Ctrl Pts',(177.8,126.297687701072,-107.75));
#20977=CARTESIAN_POINT('Ctrl Pts',(177.8,126.2,-107.75));
#20978=CARTESIAN_POINT('',(177.,127.,-106.867705939749));
#20979=CARTESIAN_POINT('Ctrl Pts',(177.,127.,-106.867705939749));
#20980=CARTESIAN_POINT('Ctrl Pts',(177.000168736525,127.,-106.867872698805));
#20981=CARTESIAN_POINT('Ctrl Pts',(177.000340729475,126.999999960859,-106.868042672762));
#20982=CARTESIAN_POINT('Ctrl Pts',(177.000571968418,126.999999795533,-106.868271119852));
#20983=CARTESIAN_POINT('Ctrl Pts',(177.000827169104,126.999999613074,-106.868523239385));
#20984=CARTESIAN_POINT('Ctrl Pts',(177.00115445911,126.99999928102,-106.868846507485));
#20985=CARTESIAN_POINT('Ctrl Pts',(177.001581551272,126.999998436683,-106.869268262893));
#20986=CARTESIAN_POINT('Ctrl Pts',(177.002058527665,126.999997493728,-106.869739279202));
#20987=CARTESIAN_POINT('Ctrl Pts',(177.002659504952,126.999995895344,-106.870332661821));
#20988=CARTESIAN_POINT('Ctrl Pts',(177.003370507335,126.999992899769,-106.871034596213));
#20989=CARTESIAN_POINT('Ctrl Pts',(177.004269736312,126.999989111163,-106.871922356591));
#20990=CARTESIAN_POINT('Ctrl Pts',(177.005343532233,126.999982983391,-106.872982343061));
#20991=CARTESIAN_POINT('Ctrl Pts',(177.006495471841,126.999973630094,-106.874119373637));
#20992=CARTESIAN_POINT('Ctrl Pts',(177.007658170838,126.999964189434,-106.875267024348));
#20993=CARTESIAN_POINT('Ctrl Pts',(177.008895009794,126.999951463521,-106.876487764087));
#20994=CARTESIAN_POINT('Ctrl Pts',(177.010105362763,126.999936173481,-106.877682323415));
#20995=CARTESIAN_POINT('Ctrl Pts',(177.011011735643,126.999924723534,-106.878576869225));
#20996=CARTESIAN_POINT('Ctrl Pts',(177.011902720356,126.999911911841,-106.879456205747));
#20997=CARTESIAN_POINT('Ctrl Pts',(177.012763689538,126.999898173663,-106.880305951649));
#20998=CARTESIAN_POINT('Ctrl Pts',(177.013545386333,126.999885700406,-106.88107745853));
#20999=CARTESIAN_POINT('Ctrl Pts',(177.014301945281,126.999872502733,-106.881824182398));
#21000=CARTESIAN_POINT('Ctrl Pts',(177.01505431964,126.999858342121,-106.882566882091));
#21001=CARTESIAN_POINT('Ctrl Pts',(177.01584139004,126.999843528486,-106.883343831674));
#21002=CARTESIAN_POINT('Ctrl Pts',(177.016631142467,126.99982752742,-106.88412355571));
#21003=CARTESIAN_POINT('Ctrl Pts',(177.017448577774,126.999809694323,-106.88493080553));
#21004=CARTESIAN_POINT('Ctrl Pts',(177.018361167524,126.999789785346,-106.885832024142));
#21005=CARTESIAN_POINT('Ctrl Pts',(177.019307696952,126.999767552882,-106.88676699424));
#21006=CARTESIAN_POINT('Ctrl Pts',(177.020269575134,126.999743173978,-106.887717360133));
#21007=CARTESIAN_POINT('Ctrl Pts',(177.021527028359,126.999711303693,-106.888959763465));
#21008=CARTESIAN_POINT('Ctrl Pts',(177.02280899112,126.999675666215,-106.890226781854));
#21009=CARTESIAN_POINT('Ctrl Pts',(177.024000600934,126.999639900927,-106.891404811913));
#21010=CARTESIAN_POINT('Ctrl Pts',(177.024974456459,126.999610671373,-106.892367569242));
#21011=CARTESIAN_POINT('Ctrl Pts',(177.025884701841,126.999581516184,-106.893267661283));
#21012=CARTESIAN_POINT('Ctrl Pts',(177.026670911014,126.999555290462,-106.894045268365));
#21013=CARTESIAN_POINT('Ctrl Pts',(177.027355513698,126.999532454046,-106.894722380656));
#21014=CARTESIAN_POINT('Ctrl Pts',(177.027945163427,126.999511912239,-106.895305724143));
#21015=CARTESIAN_POINT('Ctrl Pts',(177.028424413854,126.999494873465,-106.895779966782));
#21016=CARTESIAN_POINT('Ctrl Pts',(177.028867379516,126.999479124722,-106.896218303804));
#21017=CARTESIAN_POINT('Ctrl Pts',(177.029215532932,126.999466401456,-106.896562942416));
#21018=CARTESIAN_POINT('Ctrl Pts',(177.02948815114,126.999456345864,-106.896832907358));
#21019=CARTESIAN_POINT('Ctrl Pts',(177.029741435771,126.999447003396,-106.897083726888));
#21020=CARTESIAN_POINT('Ctrl Pts',(177.029929301386,126.999439970325,-106.897269873308));
#21021=CARTESIAN_POINT('Ctrl Pts',(177.030100163957,126.999433537031,-106.897439207673));
#21022=CARTESIAN_POINT('Ctrl Pts',(177.030133469423,126.999432283018,-106.897472215253));
#21023=CARTESIAN_POINT('Ctrl Pts',(177.030166241246,126.999431047036,-106.897504695245));
#21024=CARTESIAN_POINT('Ctrl Pts',(177.030199008002,126.999429809249,-106.897537170301));
#21025=CARTESIAN_POINT('',(177.,127.,6.35000000000001));
#21026=CARTESIAN_POINT('Origin',(177.8,122.2375,44.45));
#21027=CARTESIAN_POINT('',(177.8,123.0375,-107.75));
#21028=CARTESIAN_POINT('',(177.8,123.0375,6.35000000000001));
#21029=CARTESIAN_POINT('',(177.8,122.2375,-107.75));
#21030=CARTESIAN_POINT('Origin',(177.,123.0375,6.35000000000001));
#21031=CARTESIAN_POINT('',(177.,122.2375,-106.867705939749));
#21032=CARTESIAN_POINT('',(177.,122.2375,6.35000000000001));
#21033=CARTESIAN_POINT('',(177.030199008002,122.238070190751,-106.897537170301));
#21034=CARTESIAN_POINT('Ctrl Pts',(177.030199008002,122.238070190751,-106.897537170301));
#21035=CARTESIAN_POINT('Ctrl Pts',(177.030030585505,122.238063828476,-106.897370247161));
#21036=CARTESIAN_POINT('Ctrl Pts',(177.029858909386,122.238057382362,-106.897200107149));
#21037=CARTESIAN_POINT('Ctrl Pts',(177.029628057339,122.23804882687,-106.896971463311));
#21038=CARTESIAN_POINT('Ctrl Pts',(177.029373282892,122.238039384803,-106.896719125902));
#21039=CARTESIAN_POINT('Ctrl Pts',(177.029046504163,122.238027372131,-106.896395602126));
#21040=CARTESIAN_POINT('Ctrl Pts',(177.028620026165,122.238012105093,-106.895973543409));
#21041=CARTESIAN_POINT('Ctrl Pts',(177.0281437326,122.237995054761,-106.895502185326));
#21042=CARTESIAN_POINT('Ctrl Pts',(177.027543563761,122.237973979824,-106.894908400156));
#21043=CARTESIAN_POINT('Ctrl Pts',(177.026833440411,122.237950147598,-106.894206022241));
#21044=CARTESIAN_POINT('Ctrl Pts',(177.025935290825,122.237920005083,-106.893317668924));
#21045=CARTESIAN_POINT('Ctrl Pts',(177.0248626695,122.237885609635,-106.892257012151));
#21046=CARTESIAN_POINT('Ctrl Pts',(177.023711822739,122.237851483799,-106.891119331008));
#21047=CARTESIAN_POINT('Ctrl Pts',(177.02255032393,122.2378170421,-106.889971119675));
#21048=CARTESIAN_POINT('Ctrl Pts',(177.021314608223,122.237783080562,-106.888749855389));
#21049=CARTESIAN_POINT('Ctrl Pts',(177.02010513109,122.237752675088,-106.887554886453));
#21050=CARTESIAN_POINT('Ctrl Pts',(177.019199401769,122.237729905638,-106.886660021744));
#21051=CARTESIAN_POINT('Ctrl Pts',(177.018308923963,122.237709074602,-106.885780431506));
#21052=CARTESIAN_POINT('Ctrl Pts',(177.01744828861,122.237690299368,-106.884930519969));
#21053=CARTESIAN_POINT('Ctrl Pts',(177.016666887982,122.237673252684,-106.884158855865));
#21054=CARTESIAN_POINT('Ctrl Pts',(177.015910483884,122.237657876347,-106.883412048069));
#21055=CARTESIAN_POINT('Ctrl Pts',(177.015158111372,122.237643618104,-106.882669339888));
#21056=CARTESIAN_POINT('Ctrl Pts',(177.014371053406,122.237628702536,-106.881892391791));
#21057=CARTESIAN_POINT('Ctrl Pts',(177.013581145558,122.237614869895,-106.881112751603));
#21058=CARTESIAN_POINT('Ctrl Pts',(177.012763400083,122.237601821718,-106.880305665967));
#21059=CARTESIAN_POINT('Ctrl Pts',(177.011850452579,122.237587254471,-106.879404619322));
#21060=CARTESIAN_POINT('Ctrl Pts',(177.010903370157,122.237573726381,-106.878469920094));
#21061=CARTESIAN_POINT('Ctrl Pts',(177.009940788518,122.237561764432,-106.877519896452));
#21062=CARTESIAN_POINT('Ctrl Pts',(177.008682347608,122.237546125856,-106.876277873367));
#21063=CARTESIAN_POINT('Ctrl Pts',(177.007399134233,122.237533328235,-106.875011353485));
#21064=CARTESIAN_POINT('Ctrl Pts',(177.006206223395,122.237524073618,-106.873833867007));
#21065=CARTESIAN_POINT('Ctrl Pts',(177.005231427341,122.237516511138,-106.872871675083));
#21066=CARTESIAN_POINT('Ctrl Pts',(177.004320197307,122.237511277906,-106.871972161594));
#21067=CARTESIAN_POINT('Ctrl Pts',(177.003533069744,122.237507801652,-106.871195084158));
#21068=CARTESIAN_POINT('Ctrl Pts',(177.00284764934,122.237504774575,-106.870518415274));
#21069=CARTESIAN_POINT('Ctrl Pts',(177.002257239436,122.237503040519,-106.869935482439));
#21070=CARTESIAN_POINT('Ctrl Pts',(177.001777334963,122.237501974327,-106.869461595743));
#21071=CARTESIAN_POINT('Ctrl Pts',(177.001333761302,122.237500988851,-106.869023584289));
#21072=CARTESIAN_POINT('Ctrl Pts',(177.000985093099,122.237500559908,-106.868679225686));
#21073=CARTESIAN_POINT('Ctrl Pts',(177.000712044088,122.237500316879,-106.868409497869));
#21074=CARTESIAN_POINT('Ctrl Pts',(177.000458357708,122.237500091084,-106.868158897168));
#21075=CARTESIAN_POINT('Ctrl Pts',(177.00027016379,122.237500027304,-106.867972933222));
#21076=CARTESIAN_POINT('Ctrl Pts',(177.000098987774,122.237500006124,-106.86780376677));
#21077=CARTESIAN_POINT('Ctrl Pts',(177.000065634445,122.237500001997,-106.867770805001));
#21078=CARTESIAN_POINT('Ctrl Pts',(177.000032814728,122.2375,-106.867738369912));
#21079=CARTESIAN_POINT('Ctrl Pts',(177.,122.2375,-106.867705939749));
#21080=CARTESIAN_POINT('Ctrl Pts',(177.8,123.0375,-107.75));
#21081=CARTESIAN_POINT('Ctrl Pts',(177.8,122.939812298928,-107.75));
#21082=CARTESIAN_POINT('Ctrl Pts',(177.76680186335,122.739691653929,-107.703931901455));
#21083=CARTESIAN_POINT('Ctrl Pts',(177.539138333658,122.385326746311,-107.42587289798));
#21084=CARTESIAN_POINT('Ctrl Pts',(177.227870706314,122.245537374399,-107.093449124647));
#21085=CARTESIAN_POINT('Ctrl Pts',(177.030199008002,122.238070190751,-106.897537170301));
#21086=CARTESIAN_POINT('Origin',(139.7,122.2375,-31.75));
#21087=CARTESIAN_POINT('',(102.682294060251,122.2375,43.65));
#21088=CARTESIAN_POINT('',(120.65,122.2375,43.65));
#21089=CARTESIAN_POINT('',(102.4,122.2375,43.3677059397485));
#21090=CARTESIAN_POINT('',(102.541147030126,122.2375,43.5088529698743));
#21091=CARTESIAN_POINT('',(102.4,122.2375,-106.867705939749));
#21092=CARTESIAN_POINT('',(102.4,122.2375,-69.85));
#21093=CARTESIAN_POINT('',(102.682294060251,122.2375,-107.15));
#21094=CARTESIAN_POINT('',(102.541147030126,122.2375,-107.008852969874));
#21095=CARTESIAN_POINT('',(176.717705939749,122.2375,-107.15));
#21096=CARTESIAN_POINT('',(158.75,122.2375,-107.15));
#21097=CARTESIAN_POINT('',(176.858852969874,122.2375,-107.008852969874));
#21098=CARTESIAN_POINT('Ctrl Pts',(177.030199008002,126.999429809249,-106.897537170301));
#21099=CARTESIAN_POINT('Ctrl Pts',(177.028516554556,126.999493365079,-106.895869694655));
#21100=CARTESIAN_POINT('Ctrl Pts',(177.016175572427,126.999932103249,-106.883668236945));
#21101=CARTESIAN_POINT('Ctrl Pts',(177.002608645735,126.99999591837,-106.870285389319));
#21102=CARTESIAN_POINT('Ctrl Pts',(177.000421407138,127.,-106.868122408304));
#21103=CARTESIAN_POINT('Ctrl Pts',(177.,127.,-106.867705939749));
#21104=CARTESIAN_POINT('Ctrl Pts',(176.935978395435,126.999429809249,-106.991757782868));
#21105=CARTESIAN_POINT('Ctrl Pts',(176.934300934589,126.999493365079,-106.990085314622));
#21106=CARTESIAN_POINT('Ctrl Pts',(176.92201328382,126.999932103249,-106.977830525551));
#21107=CARTESIAN_POINT('Ctrl Pts',(176.908498481157,126.99999591837,-106.964395553897));
#21108=CARTESIAN_POINT('Ctrl Pts',(176.90632174086,127.,-106.962222074582));
#21109=CARTESIAN_POINT('Ctrl Pts',(176.905901979916,127.,-106.961803959832));
#21110=CARTESIAN_POINT('Ctrl Pts',(176.841757782868,126.999429809249,-107.085978395435));
#21111=CARTESIAN_POINT('Ctrl Pts',(176.840085314622,126.999493365079,-107.084300934589));
#21112=CARTESIAN_POINT('Ctrl Pts',(176.827830525552,127.000007709825,-107.071972508603));
#21113=CARTESIAN_POINT('Ctrl Pts',(176.814395553897,126.999950502472,-107.058492828924));
#21114=CARTESIAN_POINT('Ctrl Pts',(176.812222074582,127.,-107.05632174086));
#21115=CARTESIAN_POINT('Ctrl Pts',(176.811803959832,127.,-107.055901979916));
#21116=CARTESIAN_POINT('Ctrl Pts',(176.747537170301,126.999429809249,-107.180199008002));
#21117=CARTESIAN_POINT('Ctrl Pts',(176.745869694655,126.999493365079,-107.178516554556));
#21118=CARTESIAN_POINT('Ctrl Pts',(176.733668236945,126.999932103249,-107.166175572427));
#21119=CARTESIAN_POINT('Ctrl Pts',(176.720285389319,126.99999591837,-107.152608645735));
#21120=CARTESIAN_POINT('Ctrl Pts',(176.718122408304,127.,-107.150421407138));
#21121=CARTESIAN_POINT('Ctrl Pts',(176.717705939749,127.,-107.15));
#21122=CARTESIAN_POINT('',(176.747537170301,126.999429809249,-107.180199008002));
#21123=CARTESIAN_POINT('Ctrl Pts',(176.747537170301,126.999429809249,-107.180199008002));
#21124=CARTESIAN_POINT('Ctrl Pts',(176.841757782868,126.999429809249,-107.085978395435));
#21125=CARTESIAN_POINT('Ctrl Pts',(176.935978395435,126.999429809249,-106.991757782868));
#21126=CARTESIAN_POINT('Ctrl Pts',(177.030199008002,126.999429809249,-106.897537170301));
#21127=CARTESIAN_POINT('',(176.717705939749,127.,-107.15));
#21128=CARTESIAN_POINT('Ctrl Pts',(176.747537170301,126.999429809249,-107.180199008002));
#21129=CARTESIAN_POINT('Ctrl Pts',(176.747370247161,126.999436171524,-107.180030585505));
#21130=CARTESIAN_POINT('Ctrl Pts',(176.747200107149,126.999442617638,-107.179858909386));
#21131=CARTESIAN_POINT('Ctrl Pts',(176.746971463311,126.99945117313,-107.179628057339));
#21132=CARTESIAN_POINT('Ctrl Pts',(176.746719125902,126.999460615197,-107.179373282892));
#21133=CARTESIAN_POINT('Ctrl Pts',(176.746395602126,126.999472627869,-107.179046504163));
#21134=CARTESIAN_POINT('Ctrl Pts',(176.745973543409,126.999487894907,-107.178620026165));
#21135=CARTESIAN_POINT('Ctrl Pts',(176.745502185327,126.999504945239,-107.1781437326));
#21136=CARTESIAN_POINT('Ctrl Pts',(176.744908400156,126.999526020176,-107.177543563761));
#21137=CARTESIAN_POINT('Ctrl Pts',(176.744206022241,126.999549852402,-107.176833440411));
#21138=CARTESIAN_POINT('Ctrl Pts',(176.743317668923,126.999579994917,-107.175935290825));
#21139=CARTESIAN_POINT('Ctrl Pts',(176.742257012151,126.999614390365,-107.1748626695));
#21140=CARTESIAN_POINT('Ctrl Pts',(176.741119331007,126.999648516201,-107.173711822738));
#21141=CARTESIAN_POINT('Ctrl Pts',(176.739971119675,126.9996829579,-107.17255032393));
#21142=CARTESIAN_POINT('Ctrl Pts',(176.738749855389,126.999716919438,-107.171314608223));
#21143=CARTESIAN_POINT('Ctrl Pts',(176.737554886453,126.999747324912,-107.17010513109));
#21144=CARTESIAN_POINT('Ctrl Pts',(176.736660021744,126.999770094362,-107.169199401769));
#21145=CARTESIAN_POINT('Ctrl Pts',(176.735780431506,126.999790925398,-107.168308923963));
#21146=CARTESIAN_POINT('Ctrl Pts',(176.734930519969,126.999809700632,-107.167448288609));
#21147=CARTESIAN_POINT('Ctrl Pts',(176.734158855869,126.999826747316,-107.166666887985));
#21148=CARTESIAN_POINT('Ctrl Pts',(176.733412048076,126.999842123653,-107.165910483891));
#21149=CARTESIAN_POINT('Ctrl Pts',(176.732669339899,126.999856381896,-107.165158111383));
#21150=CARTESIAN_POINT('Ctrl Pts',(176.731892391803,126.999871297464,-107.164371053417));
#21151=CARTESIAN_POINT('Ctrl Pts',(176.731112751615,126.999885130105,-107.16358114557));
#21152=CARTESIAN_POINT('Ctrl Pts',(176.730305665979,126.999898178281,-107.162763400095));
#21153=CARTESIAN_POINT('Ctrl Pts',(176.729404619336,126.999912745528,-107.161850452592));
#21154=CARTESIAN_POINT('Ctrl Pts',(176.728469920108,126.999926273619,-107.160903370172));
#21155=CARTESIAN_POINT('Ctrl Pts',(176.727519896467,126.999938235568,-107.159940788534));
#21156=CARTESIAN_POINT('Ctrl Pts',(176.726277873387,126.999953874144,-107.158682347629));
#21157=CARTESIAN_POINT('Ctrl Pts',(176.72501135351,126.999966671765,-107.157399134258));
#21158=CARTESIAN_POINT('Ctrl Pts',(176.723833867035,126.999975926382,-107.156206223424));
#21159=CARTESIAN_POINT('Ctrl Pts',(176.722871675108,126.999983488862,-107.155231427366));
#21160=CARTESIAN_POINT('Ctrl Pts',(176.721972161615,126.999988722094,-107.154320197329));
#21161=CARTESIAN_POINT('Ctrl Pts',(176.721195084176,126.999992198348,-107.153533069762));
#21162=CARTESIAN_POINT('Ctrl Pts',(176.72051841529,126.999995225425,-107.152847649357));
#21163=CARTESIAN_POINT('Ctrl Pts',(176.719935482452,126.999996959481,-107.15225723945));
#21164=CARTESIAN_POINT('Ctrl Pts',(176.719461595755,126.999998025673,-107.151777334975));
#21165=CARTESIAN_POINT('Ctrl Pts',(176.719023584299,126.999999011149,-107.151333761312));
#21166=CARTESIAN_POINT('Ctrl Pts',(176.718679225694,126.999999440092,-107.150985093108));
#21167=CARTESIAN_POINT('Ctrl Pts',(176.718409497876,126.999999683121,-107.150712044095));
#21168=CARTESIAN_POINT('Ctrl Pts',(176.718158897173,126.999999908916,-107.150458357714));
#21169=CARTESIAN_POINT('Ctrl Pts',(176.717972933227,126.999999972695,-107.150270163795));
#21170=CARTESIAN_POINT('Ctrl Pts',(176.717803766775,126.999999993876,-107.150098987779));
#21171=CARTESIAN_POINT('Ctrl Pts',(176.717770805004,126.999999998003,-107.150065634448));
#21172=CARTESIAN_POINT('Ctrl Pts',(176.717738369913,127.,-107.150032814729));
#21173=CARTESIAN_POINT('Ctrl Pts',(176.717705939749,127.,-107.15));
#21174=CARTESIAN_POINT('',(176.858852969874,127.,-107.008852969874));
#21175=CARTESIAN_POINT('Ctrl Pts',(176.747537170301,122.238070190751,-107.180199008002));
#21176=CARTESIAN_POINT('Ctrl Pts',(176.745869694655,122.238006634921,-107.178516554556));
#21177=CARTESIAN_POINT('Ctrl Pts',(176.733668171844,122.237567895484,-107.16617550697));
#21178=CARTESIAN_POINT('Ctrl Pts',(176.720285372322,122.237504081409,-107.152608628619));
#21179=CARTESIAN_POINT('Ctrl Pts',(176.718122408304,122.2375,-107.150421407138));
#21180=CARTESIAN_POINT('Ctrl Pts',(176.717705939749,122.2375,-107.15));
#21181=CARTESIAN_POINT('Ctrl Pts',(176.841757782868,122.238070190751,-107.085978395435));
#21182=CARTESIAN_POINT('Ctrl Pts',(176.840085314622,122.238006634921,-107.084300934589));
#21183=CARTESIAN_POINT('Ctrl Pts',(176.82783046045,122.237567895484,-107.072013218364));
#21184=CARTESIAN_POINT('Ctrl Pts',(176.8143955369,122.237504081409,-107.058498464041));
#21185=CARTESIAN_POINT('Ctrl Pts',(176.812222074582,122.2375,-107.05632174086));
#21186=CARTESIAN_POINT('Ctrl Pts',(176.811803959832,122.2375,-107.055901979916));
#21187=CARTESIAN_POINT('Ctrl Pts',(176.935978395435,122.238070190751,-106.991757782868));
#21188=CARTESIAN_POINT('Ctrl Pts',(176.934300934589,122.238006634921,-106.990085314622));
#21189=CARTESIAN_POINT('Ctrl Pts',(176.921972442847,122.237492296595,-106.97783046045));
#21190=CARTESIAN_POINT('Ctrl Pts',(176.908492811756,122.237549499319,-106.9643955369));
#21191=CARTESIAN_POINT('Ctrl Pts',(176.90632174086,122.2375,-106.962222074582));
#21192=CARTESIAN_POINT('Ctrl Pts',(176.905901979916,122.2375,-106.961803959832));
#21193=CARTESIAN_POINT('Ctrl Pts',(177.030199008002,122.238070190751,-106.897537170301));
#21194=CARTESIAN_POINT('Ctrl Pts',(177.028516554556,122.238006634921,-106.895869694655));
#21195=CARTESIAN_POINT('Ctrl Pts',(177.01617550697,122.237567895484,-106.883668171843));
#21196=CARTESIAN_POINT('Ctrl Pts',(177.002608628619,122.237504081409,-106.870285372322));
#21197=CARTESIAN_POINT('Ctrl Pts',(177.000421407138,122.2375,-106.868122408304));
#21198=CARTESIAN_POINT('Ctrl Pts',(177.,122.2375,-106.867705939749));
#21199=CARTESIAN_POINT('',(176.747537170301,122.238070190751,-107.180199008002));
#21200=CARTESIAN_POINT('Ctrl Pts',(176.717705939749,122.2375,-107.15));
#21201=CARTESIAN_POINT('Ctrl Pts',(176.717872698805,122.2375,-107.150168736525));
#21202=CARTESIAN_POINT('Ctrl Pts',(176.718042672762,122.237500039141,-107.150340729475));
#21203=CARTESIAN_POINT('Ctrl Pts',(176.718271119852,122.237500204467,-107.150571968418));
#21204=CARTESIAN_POINT('Ctrl Pts',(176.718523239385,122.237500386926,-107.150827169104));
#21205=CARTESIAN_POINT('Ctrl Pts',(176.718846507485,122.23750071898,-107.15115445911));
#21206=CARTESIAN_POINT('Ctrl Pts',(176.719268262893,122.237501563317,-107.151581551272));
#21207=CARTESIAN_POINT('Ctrl Pts',(176.719739279202,122.237502506272,-107.152058527665));
#21208=CARTESIAN_POINT('Ctrl Pts',(176.720332661821,122.237504104656,-107.152659504951));
#21209=CARTESIAN_POINT('Ctrl Pts',(176.721034596213,122.237507100231,-107.153370507335));
#21210=CARTESIAN_POINT('Ctrl Pts',(176.721922356591,122.237510888837,-107.154269736312));
#21211=CARTESIAN_POINT('Ctrl Pts',(176.72298234306,122.237517016609,-107.155343532233));
#21212=CARTESIAN_POINT('Ctrl Pts',(176.724119373636,122.237526369906,-107.15649547184));
#21213=CARTESIAN_POINT('Ctrl Pts',(176.725267024347,122.237535810566,-107.157658170837));
#21214=CARTESIAN_POINT('Ctrl Pts',(176.726487764087,122.237548536479,-107.158895009794));
#21215=CARTESIAN_POINT('Ctrl Pts',(176.727682323414,122.237563826519,-107.160105362763));
#21216=CARTESIAN_POINT('Ctrl Pts',(176.728576869224,122.237575276466,-107.161011735642));
#21217=CARTESIAN_POINT('Ctrl Pts',(176.729456205746,122.237588088159,-107.161902720355));
#21218=CARTESIAN_POINT('Ctrl Pts',(176.730305951649,122.237601826337,-107.162763689537));
#21219=CARTESIAN_POINT('Ctrl Pts',(176.731077458528,122.237614299594,-107.16354538633));
#21220=CARTESIAN_POINT('Ctrl Pts',(176.731824182394,122.237627497267,-107.164301945277));
#21221=CARTESIAN_POINT('Ctrl Pts',(176.732566882086,122.237641657879,-107.165054319635));
#21222=CARTESIAN_POINT('Ctrl Pts',(176.733343831668,122.237656471514,-107.165841390034));
#21223=CARTESIAN_POINT('Ctrl Pts',(176.734123555703,122.23767247258,-107.166631142461));
#21224=CARTESIAN_POINT('Ctrl Pts',(176.734930805524,122.237690305676,-107.167448577767));
#21225=CARTESIAN_POINT('Ctrl Pts',(176.735832024135,122.237710214654,-107.168361167517));
#21226=CARTESIAN_POINT('Ctrl Pts',(176.736766994232,122.237732447118,-107.169307696944));
#21227=CARTESIAN_POINT('Ctrl Pts',(176.737717360126,122.237756826022,-107.170269575126));
#21228=CARTESIAN_POINT('Ctrl Pts',(176.738959763455,122.237788696307,-107.171527028349));
#21229=CARTESIAN_POINT('Ctrl Pts',(176.740226781842,122.237824333784,-107.172808991109));
#21230=CARTESIAN_POINT('Ctrl Pts',(176.741404811901,122.237860099072,-107.174000600922));
#21231=CARTESIAN_POINT('Ctrl Pts',(176.742367569231,122.237889328627,-107.174974456448));
#21232=CARTESIAN_POINT('Ctrl Pts',(176.743267661274,122.237918483816,-107.175884701832));
#21233=CARTESIAN_POINT('Ctrl Pts',(176.744045268357,122.237944709538,-107.176670911006));
#21234=CARTESIAN_POINT('Ctrl Pts',(176.74472238065,122.237967545954,-107.17735551369));
#21235=CARTESIAN_POINT('Ctrl Pts',(176.745305724137,122.237988087761,-107.177945163421));
#21236=CARTESIAN_POINT('Ctrl Pts',(176.745779966777,122.238005126535,-107.178424413848));
#21237=CARTESIAN_POINT('Ctrl Pts',(176.7462183038,122.238020875278,-107.178867379512));
#21238=CARTESIAN_POINT('Ctrl Pts',(176.746562942412,122.238033598544,-107.179215532928));
#21239=CARTESIAN_POINT('Ctrl Pts',(176.746832907355,122.238043654136,-107.179488151137));
#21240=CARTESIAN_POINT('Ctrl Pts',(176.747083726886,122.238052996604,-107.179741435769));
#21241=CARTESIAN_POINT('Ctrl Pts',(176.747269873306,122.238060029674,-107.179929301384));
#21242=CARTESIAN_POINT('Ctrl Pts',(176.747439207671,122.238066462969,-107.180100163954));
#21243=CARTESIAN_POINT('Ctrl Pts',(176.747472215252,122.238067716982,-107.180133469422));
#21244=CARTESIAN_POINT('Ctrl Pts',(176.747504695245,122.238068952964,-107.180166241245));
#21245=CARTESIAN_POINT('Ctrl Pts',(176.747537170301,122.238070190751,-107.180199008002));
#21246=CARTESIAN_POINT('Ctrl Pts',(177.030199008002,122.238070190751,-106.897537170301));
#21247=CARTESIAN_POINT('Ctrl Pts',(176.935978395435,122.238070190751,-106.991757782868));
#21248=CARTESIAN_POINT('Ctrl Pts',(176.841757782868,122.238070190751,-107.085978395435));
#21249=CARTESIAN_POINT('Ctrl Pts',(176.747537170301,122.238070190751,-107.180199008002));
#21250=CARTESIAN_POINT('Ctrl Pts',(177.030199008002,122.238070190751,-106.897537170301));
#21251=CARTESIAN_POINT('Ctrl Pts',(177.227870706314,122.245537374399,-107.093449124647));
#21252=CARTESIAN_POINT('Ctrl Pts',(177.539138333658,122.385326746311,-107.42587289798));
#21253=CARTESIAN_POINT('Ctrl Pts',(177.76680186335,122.739691653929,-107.703931901455));
#21254=CARTESIAN_POINT('Ctrl Pts',(177.8,122.939812298928,-107.75));
#21255=CARTESIAN_POINT('Ctrl Pts',(177.8,123.0375,-107.75));
#21256=CARTESIAN_POINT('Ctrl Pts',(176.935978395435,122.238070190751,-106.991757782868));
#21257=CARTESIAN_POINT('Ctrl Pts',(177.133063512425,122.245537374399,-107.188256318536));
#21258=CARTESIAN_POINT('Ctrl Pts',(177.451383188432,122.385326746311,-107.513628043206));
#21259=CARTESIAN_POINT('Ctrl Pts',(177.695845209385,122.739691653929,-107.77488855542));
#21260=CARTESIAN_POINT('Ctrl Pts',(177.733333333333,122.939812298928,-107.816666666667));
#21261=CARTESIAN_POINT('Ctrl Pts',(177.733333333333,123.0375,-107.816666666667));
#21262=CARTESIAN_POINT('Ctrl Pts',(176.841757782868,122.238070190751,-107.085978395435));
#21263=CARTESIAN_POINT('Ctrl Pts',(177.038256318536,122.245537374399,-107.283063512425));
#21264=CARTESIAN_POINT('Ctrl Pts',(177.363628043206,122.385326746311,-107.601383188432));
#21265=CARTESIAN_POINT('Ctrl Pts',(177.62488855542,122.739691653929,-107.845845209385));
#21266=CARTESIAN_POINT('Ctrl Pts',(177.666666666667,122.939812298928,-107.883333333333));
#21267=CARTESIAN_POINT('Ctrl Pts',(177.666666666667,123.0375,-107.883333333333));
#21268=CARTESIAN_POINT('Ctrl Pts',(176.747537170301,122.238070190751,-107.180199008002));
#21269=CARTESIAN_POINT('Ctrl Pts',(176.943449124647,122.245537374399,-107.377870706314));
#21270=CARTESIAN_POINT('Ctrl Pts',(177.27587289798,122.385326746311,-107.689138333658));
#21271=CARTESIAN_POINT('Ctrl Pts',(177.553931901455,122.739691653929,-107.91680186335));
#21272=CARTESIAN_POINT('Ctrl Pts',(177.6,122.939812298928,-107.95));
#21273=CARTESIAN_POINT('Ctrl Pts',(177.6,123.0375,-107.95));
#21274=CARTESIAN_POINT('',(177.6,123.0375,-107.95));
#21275=CARTESIAN_POINT('Ctrl Pts',(176.747537170301,122.238070190751,-107.180199008002));
#21276=CARTESIAN_POINT('Ctrl Pts',(176.943449124647,122.245537374399,-107.377870706314));
#21277=CARTESIAN_POINT('Ctrl Pts',(177.27587289798,122.385326746311,-107.689138333658));
#21278=CARTESIAN_POINT('Ctrl Pts',(177.553931901455,122.739691653929,-107.91680186335));
#21279=CARTESIAN_POINT('Ctrl Pts',(177.6,122.939812298928,-107.95));
#21280=CARTESIAN_POINT('Ctrl Pts',(177.6,123.0375,-107.95));
#21281=CARTESIAN_POINT('',(177.6,123.0375,-107.95));
#21282=CARTESIAN_POINT('Origin',(177.7,122.2375,-107.85));
#21283=CARTESIAN_POINT('',(177.6,126.2,-107.95));
#21284=CARTESIAN_POINT('',(177.6,126.2,-107.95));
#21285=CARTESIAN_POINT('',(177.6,122.2375,-107.95));
#21286=CARTESIAN_POINT('Ctrl Pts',(176.747537170301,126.999429809249,-107.180199008002));
#21287=CARTESIAN_POINT('Ctrl Pts',(176.943449124647,126.991962625601,-107.377870706314));
#21288=CARTESIAN_POINT('Ctrl Pts',(177.275873068733,126.852173302019,-107.689138426476));
#21289=CARTESIAN_POINT('Ctrl Pts',(177.553932070819,126.49780856488,-107.916802032304));
#21290=CARTESIAN_POINT('Ctrl Pts',(177.6,126.297687701072,-107.95));
#21291=CARTESIAN_POINT('Ctrl Pts',(177.6,126.2,-107.95));
#21292=CARTESIAN_POINT('Ctrl Pts',(176.841757782868,126.999429809249,-107.085978395435));
#21293=CARTESIAN_POINT('Ctrl Pts',(177.038256318536,126.991962625601,-107.283063512425));
#21294=CARTESIAN_POINT('Ctrl Pts',(177.363628187981,126.852173302019,-107.601383307228));
#21295=CARTESIAN_POINT('Ctrl Pts',(177.624888724647,126.49780856488,-107.845845378476));
#21296=CARTESIAN_POINT('Ctrl Pts',(177.666666666667,126.297687701072,-107.883333333333));
#21297=CARTESIAN_POINT('Ctrl Pts',(177.666666666667,126.2,-107.883333333333));
#21298=CARTESIAN_POINT('Ctrl Pts',(176.935978395435,126.999429809249,-106.991757782868));
#21299=CARTESIAN_POINT('Ctrl Pts',(177.133063512425,126.991962625601,-107.188256318536));
#21300=CARTESIAN_POINT('Ctrl Pts',(177.451383307228,126.852173302019,-107.513628187981));
#21301=CARTESIAN_POINT('Ctrl Pts',(177.695845378476,126.49780856488,-107.774888724647));
#21302=CARTESIAN_POINT('Ctrl Pts',(177.733333333333,126.297687701072,-107.816666666667));
#21303=CARTESIAN_POINT('Ctrl Pts',(177.733333333333,126.2,-107.816666666667));
#21304=CARTESIAN_POINT('Ctrl Pts',(177.030199008002,126.999429809249,-106.897537170301));
#21305=CARTESIAN_POINT('Ctrl Pts',(177.227870706314,126.991962625601,-107.093449124647));
#21306=CARTESIAN_POINT('Ctrl Pts',(177.539138426476,126.852173302019,-107.425873068733));
#21307=CARTESIAN_POINT('Ctrl Pts',(177.766802032304,126.49780856488,-107.703932070819));
#21308=CARTESIAN_POINT('Ctrl Pts',(177.8,126.297687701072,-107.75));
#21309=CARTESIAN_POINT('Ctrl Pts',(177.8,126.2,-107.75));
#21310=CARTESIAN_POINT('Ctrl Pts',(177.6,126.2,-107.95));
#21311=CARTESIAN_POINT('Ctrl Pts',(177.6,126.297687701072,-107.95));
#21312=CARTESIAN_POINT('Ctrl Pts',(177.553932070819,126.49780856488,-107.916802032304));
#21313=CARTESIAN_POINT('Ctrl Pts',(177.275873068733,126.852173302019,-107.689138426476));
#21314=CARTESIAN_POINT('Ctrl Pts',(176.943449124647,126.991962625601,-107.377870706314));
#21315=CARTESIAN_POINT('Ctrl Pts',(176.747537170301,126.999429809249,-107.180199008002));
#21316=CARTESIAN_POINT('Origin',(158.75,126.2,-107.15));
#21317=CARTESIAN_POINT('',(101.8,126.2,-107.95));
#21318=CARTESIAN_POINT('',(158.75,126.2,-107.95));
#21319=CARTESIAN_POINT('',(102.652462829699,126.999429809249,-107.180199008002));
#21320=CARTESIAN_POINT('Ctrl Pts',(102.652462829699,126.999429809249,-107.180199008002));
#21321=CARTESIAN_POINT('Ctrl Pts',(102.456550875353,126.991962625601,-107.377870706314));
#21322=CARTESIAN_POINT('Ctrl Pts',(102.124131493119,126.852172058915,-107.68913596838));
#21323=CARTESIAN_POINT('Ctrl Pts',(101.846072469497,126.49780266677,-107.916797488447));
#21324=CARTESIAN_POINT('Ctrl Pts',(101.8,126.297687701072,-107.95));
#21325=CARTESIAN_POINT('Ctrl Pts',(101.8,126.2,-107.95));
#21326=CARTESIAN_POINT('',(102.682294060251,127.,-107.15));
#21327=CARTESIAN_POINT('Ctrl Pts',(102.682294060251,127.,-107.15));
#21328=CARTESIAN_POINT('Ctrl Pts',(102.682127301195,127.,-107.150168736525));
#21329=CARTESIAN_POINT('Ctrl Pts',(102.681957327238,126.999999960859,-107.150340729475));
#21330=CARTESIAN_POINT('Ctrl Pts',(102.681728880148,126.999999795533,-107.150571968418));
#21331=CARTESIAN_POINT('Ctrl Pts',(102.681476760615,126.999999613074,-107.150827169104));
#21332=CARTESIAN_POINT('Ctrl Pts',(102.681153492515,126.99999928102,-107.15115445911));
#21333=CARTESIAN_POINT('Ctrl Pts',(102.680731737107,126.999998436683,-107.151581551272));
#21334=CARTESIAN_POINT('Ctrl Pts',(102.680260720798,126.999997493728,-107.152058527665));
#21335=CARTESIAN_POINT('Ctrl Pts',(102.679667338179,126.999995895344,-107.152659504951));
#21336=CARTESIAN_POINT('Ctrl Pts',(102.678965403787,126.999992899769,-107.153370507335));
#21337=CARTESIAN_POINT('Ctrl Pts',(102.678077643409,126.999989111163,-107.154269736312));
#21338=CARTESIAN_POINT('Ctrl Pts',(102.67701765694,126.999982983391,-107.155343532233));
#21339=CARTESIAN_POINT('Ctrl Pts',(102.675880626364,126.999973630094,-107.156495471841));
#21340=CARTESIAN_POINT('Ctrl Pts',(102.674732975653,126.999964189434,-107.157658170837));
#21341=CARTESIAN_POINT('Ctrl Pts',(102.673512235913,126.999951463521,-107.158895009794));
#21342=CARTESIAN_POINT('Ctrl Pts',(102.672317676586,126.999936173481,-107.160105362763));
#21343=CARTESIAN_POINT('Ctrl Pts',(102.671423130776,126.999924723534,-107.161011735643));
#21344=CARTESIAN_POINT('Ctrl Pts',(102.670543794253,126.999911911841,-107.161902720355));
#21345=CARTESIAN_POINT('Ctrl Pts',(102.669694048351,126.999898173663,-107.162763689538));
#21346=CARTESIAN_POINT('Ctrl Pts',(102.66892254147,126.999885700406,-107.163545386333));
#21347=CARTESIAN_POINT('Ctrl Pts',(102.668175817602,126.999872502733,-107.164301945281));
#21348=CARTESIAN_POINT('Ctrl Pts',(102.667433117909,126.999858342121,-107.16505431964));
#21349=CARTESIAN_POINT('Ctrl Pts',(102.666656168326,126.999843528486,-107.16584139004));
#21350=CARTESIAN_POINT('Ctrl Pts',(102.66587644429,126.99982752742,-107.166631142467));
#21351=CARTESIAN_POINT('Ctrl Pts',(102.66506919447,126.999809694323,-107.167448577774));
#21352=CARTESIAN_POINT('Ctrl Pts',(102.664167975858,126.999789785346,-107.168361167524));
#21353=CARTESIAN_POINT('Ctrl Pts',(102.66323300576,126.999767552882,-107.169307696952));
#21354=CARTESIAN_POINT('Ctrl Pts',(102.662282639866,126.999743173978,-107.170269575135));
#21355=CARTESIAN_POINT('Ctrl Pts',(102.661040236535,126.999711303693,-107.171527028359));
#21356=CARTESIAN_POINT('Ctrl Pts',(102.659773218146,126.999675666215,-107.172808991121));
#21357=CARTESIAN_POINT('Ctrl Pts',(102.658595188086,126.999639900927,-107.174000600935));
#21358=CARTESIAN_POINT('Ctrl Pts',(102.657632430757,126.999610671373,-107.174974456459));
#21359=CARTESIAN_POINT('Ctrl Pts',(102.656732338716,126.999581516184,-107.175884701842));
#21360=CARTESIAN_POINT('Ctrl Pts',(102.655954731635,126.999555290462,-107.176670911014));
#21361=CARTESIAN_POINT('Ctrl Pts',(102.655277619343,126.999532454046,-107.177355513698));
#21362=CARTESIAN_POINT('Ctrl Pts',(102.654694275857,126.999511912239,-107.177945163427));
#21363=CARTESIAN_POINT('Ctrl Pts',(102.654220033218,126.999494873465,-107.178424413854));
#21364=CARTESIAN_POINT('Ctrl Pts',(102.653781696196,126.999479124722,-107.178867379516));
#21365=CARTESIAN_POINT('Ctrl Pts',(102.653437057584,126.999466401456,-107.179215532932));
#21366=CARTESIAN_POINT('Ctrl Pts',(102.653167092642,126.999456345864,-107.17948815114));
#21367=CARTESIAN_POINT('Ctrl Pts',(102.652916273112,126.999447003396,-107.179741435771));
#21368=CARTESIAN_POINT('Ctrl Pts',(102.652730126692,126.999439970325,-107.179929301386));
#21369=CARTESIAN_POINT('Ctrl Pts',(102.652560792327,126.999433537031,-107.180100163956));
#21370=CARTESIAN_POINT('Ctrl Pts',(102.652527784747,126.999432283018,-107.180133469423));
#21371=CARTESIAN_POINT('Ctrl Pts',(102.652495304755,126.999431047036,-107.180166241246));
#21372=CARTESIAN_POINT('Ctrl Pts',(102.652462829699,126.999429809249,-107.180199008002));
#21373=CARTESIAN_POINT('',(158.75,127.,-107.15));
#21374=CARTESIAN_POINT('Origin',(177.8,122.2375,-107.95));
#21375=CARTESIAN_POINT('',(101.8,123.0375,-107.95));
#21376=CARTESIAN_POINT('',(158.75,123.0375,-107.95));
#21377=CARTESIAN_POINT('',(101.8,122.2375,-107.95));
#21378=CARTESIAN_POINT('Origin',(158.75,123.0375,-107.15));
#21379=CARTESIAN_POINT('',(102.652462829699,122.238070190751,-107.180199008002));
#21380=CARTESIAN_POINT('Ctrl Pts',(102.652462829699,122.238070190751,-107.180199008002));
#21381=CARTESIAN_POINT('Ctrl Pts',(102.652629752839,122.238063828476,-107.180030585505));
#21382=CARTESIAN_POINT('Ctrl Pts',(102.652799892851,122.238057382362,-107.179858909386));
#21383=CARTESIAN_POINT('Ctrl Pts',(102.653028536689,122.23804882687,-107.179628057339));
#21384=CARTESIAN_POINT('Ctrl Pts',(102.653280874098,122.238039384803,-107.179373282892));
#21385=CARTESIAN_POINT('Ctrl Pts',(102.653604397874,122.238027372131,-107.179046504163));
#21386=CARTESIAN_POINT('Ctrl Pts',(102.654026456591,122.238012105093,-107.178620026165));
#21387=CARTESIAN_POINT('Ctrl Pts',(102.654497814673,122.237995054761,-107.1781437326));
#21388=CARTESIAN_POINT('Ctrl Pts',(102.655091599844,122.237973979824,-107.177543563761));
#21389=CARTESIAN_POINT('Ctrl Pts',(102.655793977759,122.237950147598,-107.176833440411));
#21390=CARTESIAN_POINT('Ctrl Pts',(102.656682331076,122.237920005083,-107.175935290825));
#21391=CARTESIAN_POINT('Ctrl Pts',(102.657742987849,122.237885609635,-107.1748626695));
#21392=CARTESIAN_POINT('Ctrl Pts',(102.658880668992,122.237851483799,-107.173711822739));
#21393=CARTESIAN_POINT('Ctrl Pts',(102.660028880325,122.2378170421,-107.17255032393));
#21394=CARTESIAN_POINT('Ctrl Pts',(102.661250144611,122.237783080562,-107.171314608223));
#21395=CARTESIAN_POINT('Ctrl Pts',(102.662445113547,122.237752675088,-107.17010513109));
#21396=CARTESIAN_POINT('Ctrl Pts',(102.663339978256,122.237729905638,-107.169199401769));
#21397=CARTESIAN_POINT('Ctrl Pts',(102.664219568494,122.237709074602,-107.168308923963));
#21398=CARTESIAN_POINT('Ctrl Pts',(102.665069480031,122.237690299368,-107.167448288609));
#21399=CARTESIAN_POINT('Ctrl Pts',(102.665841144133,122.237673252684,-107.166666887983));
#21400=CARTESIAN_POINT('Ctrl Pts',(102.666587951927,122.237657876347,-107.165910483887));
#21401=CARTESIAN_POINT('Ctrl Pts',(102.667330660107,122.237643618104,-107.165158111378));
#21402=CARTESIAN_POINT('Ctrl Pts',(102.668107608203,122.237628702536,-107.164371053412));
#21403=CARTESIAN_POINT('Ctrl Pts',(102.668887248391,122.237614869895,-107.163581145565));
#21404=CARTESIAN_POINT('Ctrl Pts',(102.669694334027,122.237601821718,-107.162763400089));
#21405=CARTESIAN_POINT('Ctrl Pts',(102.670595380671,122.237587254472,-107.161850452586));
#21406=CARTESIAN_POINT('Ctrl Pts',(102.671530079899,122.237573726381,-107.160903370165));
#21407=CARTESIAN_POINT('Ctrl Pts',(102.67248010354,122.237561764432,-107.159940788526));
#21408=CARTESIAN_POINT('Ctrl Pts',(102.673722126622,122.237546125856,-107.158682347619));
#21409=CARTESIAN_POINT('Ctrl Pts',(102.674988646501,122.237533328235,-107.157399134247));
#21410=CARTESIAN_POINT('Ctrl Pts',(102.676166132978,122.237524073618,-107.156206223411));
#21411=CARTESIAN_POINT('Ctrl Pts',(102.677128324903,122.237516511138,-107.155231427355));
#21412=CARTESIAN_POINT('Ctrl Pts',(102.678027838394,122.237511277906,-107.154320197319));
#21413=CARTESIAN_POINT('Ctrl Pts',(102.678804915832,122.237507801652,-107.153533069754));
#21414=CARTESIAN_POINT('Ctrl Pts',(102.679481584717,122.237504774575,-107.152847649349));
#21415=CARTESIAN_POINT('Ctrl Pts',(102.680064517554,122.237503040519,-107.152257239444));
#21416=CARTESIAN_POINT('Ctrl Pts',(102.68053840425,122.237501974327,-107.151777334969));
#21417=CARTESIAN_POINT('Ctrl Pts',(102.680976415705,122.237500988851,-107.151333761308));
#21418=CARTESIAN_POINT('Ctrl Pts',(102.681320774309,122.237500559908,-107.150985093104));
#21419=CARTESIAN_POINT('Ctrl Pts',(102.681590502127,122.237500316879,-107.150712044092));
#21420=CARTESIAN_POINT('Ctrl Pts',(102.681841102829,122.237500091084,-107.150458357711));
#21421=CARTESIAN_POINT('Ctrl Pts',(102.682027066775,122.237500027304,-107.150270163793));
#21422=CARTESIAN_POINT('Ctrl Pts',(102.682196233227,122.237500006124,-107.150098987777));
#21423=CARTESIAN_POINT('Ctrl Pts',(102.682229194998,122.237500001997,-107.150065634446));
#21424=CARTESIAN_POINT('Ctrl Pts',(102.682261630087,122.2375,-107.150032814729));
#21425=CARTESIAN_POINT('Ctrl Pts',(102.682294060251,122.2375,-107.15));
#21426=CARTESIAN_POINT('Ctrl Pts',(101.8,123.0375,-107.95));
#21427=CARTESIAN_POINT('Ctrl Pts',(101.8,122.939812298928,-107.95));
#21428=CARTESIAN_POINT('Ctrl Pts',(101.84607276554,122.739697720169,-107.916797191109));
#21429=CARTESIAN_POINT('Ctrl Pts',(102.124131789418,122.385328018291,-107.689135810314));
#21430=CARTESIAN_POINT('Ctrl Pts',(102.456550875353,122.245537374399,-107.377870706314));
#21431=CARTESIAN_POINT('Ctrl Pts',(102.652462829699,122.238070190751,-107.180199008002));
#21432=CARTESIAN_POINT('Ctrl Pts',(102.369800991998,122.238070190751,-106.897537170301));
#21433=CARTESIAN_POINT('Ctrl Pts',(102.371483445444,122.238006634921,-106.895869694655));
#21434=CARTESIAN_POINT('Ctrl Pts',(102.38382574621,122.237567871227,-106.883666925463));
#21435=CARTESIAN_POINT('Ctrl Pts',(102.397391698643,122.237504077204,-106.870285047339));
#21436=CARTESIAN_POINT('Ctrl Pts',(102.399578592862,122.2375,-106.868122408304));
#21437=CARTESIAN_POINT('Ctrl Pts',(102.4,122.2375,-106.867705939749));
#21438=CARTESIAN_POINT('Ctrl Pts',(102.464021604565,122.238070190751,-106.991757782868));
#21439=CARTESIAN_POINT('Ctrl Pts',(102.465699065411,122.238006634921,-106.990085314622));
#21440=CARTESIAN_POINT('Ctrl Pts',(102.477988034816,122.237567871227,-106.977829214069));
#21441=CARTESIAN_POINT('Ctrl Pts',(102.491501863221,122.237504077204,-106.964395211916));
#21442=CARTESIAN_POINT('Ctrl Pts',(102.49367825914,122.2375,-106.962222074582));
#21443=CARTESIAN_POINT('Ctrl Pts',(102.494098020084,122.2375,-106.961803959832));
#21444=CARTESIAN_POINT('Ctrl Pts',(102.558242217132,122.238070190751,-107.085978395435));
#21445=CARTESIAN_POINT('Ctrl Pts',(102.559914685378,122.238006634921,-107.084300934589));
#21446=CARTESIAN_POINT('Ctrl Pts',(102.572170785931,122.237492419513,-107.071971183941));
#21447=CARTESIAN_POINT('Ctrl Pts',(102.585604788083,122.237549533561,-107.058492483501));
#21448=CARTESIAN_POINT('Ctrl Pts',(102.587777925418,122.2375,-107.05632174086));
#21449=CARTESIAN_POINT('Ctrl Pts',(102.588196040168,122.2375,-107.055901979916));
#21450=CARTESIAN_POINT('Ctrl Pts',(102.652462829699,122.238070190751,-107.180199008002));
#21451=CARTESIAN_POINT('Ctrl Pts',(102.654130305345,122.238006634921,-107.178516554556));
#21452=CARTESIAN_POINT('Ctrl Pts',(102.666333074537,122.237567871227,-107.16617425379));
#21453=CARTESIAN_POINT('Ctrl Pts',(102.679714952661,122.237504077204,-107.152608301357));
#21454=CARTESIAN_POINT('Ctrl Pts',(102.681877591696,122.2375,-107.150421407138));
#21455=CARTESIAN_POINT('Ctrl Pts',(102.682294060251,122.2375,-107.15));
#21456=CARTESIAN_POINT('',(102.369800991998,122.238070190751,-106.897537170301));
#21457=CARTESIAN_POINT('Ctrl Pts',(102.4,122.2375,-106.867705939749));
#21458=CARTESIAN_POINT('Ctrl Pts',(102.399831263475,122.2375,-106.867872698805));
#21459=CARTESIAN_POINT('Ctrl Pts',(102.399659270525,122.237500039141,-106.868042672762));
#21460=CARTESIAN_POINT('Ctrl Pts',(102.399428031582,122.237500204467,-106.868271119852));
#21461=CARTESIAN_POINT('Ctrl Pts',(102.399172830896,122.237500386926,-106.868523239385));
#21462=CARTESIAN_POINT('Ctrl Pts',(102.39884554089,122.23750071898,-106.868846507485));
#21463=CARTESIAN_POINT('Ctrl Pts',(102.398418448728,122.237501563317,-106.869268262893));
#21464=CARTESIAN_POINT('Ctrl Pts',(102.397941472335,122.237502506272,-106.869739279202));
#21465=CARTESIAN_POINT('Ctrl Pts',(102.397340495049,122.237504104656,-106.870332661821));
#21466=CARTESIAN_POINT('Ctrl Pts',(102.396629492665,122.237507100231,-106.871034596213));
#21467=CARTESIAN_POINT('Ctrl Pts',(102.395730263688,122.237510888837,-106.871922356591));
#21468=CARTESIAN_POINT('Ctrl Pts',(102.394656467767,122.237517016609,-106.87298234306));
#21469=CARTESIAN_POINT('Ctrl Pts',(102.39350452816,122.237526369906,-106.874119373636));
#21470=CARTESIAN_POINT('Ctrl Pts',(102.392341829163,122.237535810566,-106.875267024347));
#21471=CARTESIAN_POINT('Ctrl Pts',(102.391104990206,122.237548536479,-106.876487764087));
#21472=CARTESIAN_POINT('Ctrl Pts',(102.389894637237,122.237563826519,-106.877682323414));
#21473=CARTESIAN_POINT('Ctrl Pts',(102.388988264358,122.237575276466,-106.878576869224));
#21474=CARTESIAN_POINT('Ctrl Pts',(102.388097279645,122.237588088159,-106.879456205746));
#21475=CARTESIAN_POINT('Ctrl Pts',(102.387236310463,122.237601826337,-106.880305951649));
#21476=CARTESIAN_POINT('Ctrl Pts',(102.386454613668,122.237614299594,-106.881077458529));
#21477=CARTESIAN_POINT('Ctrl Pts',(102.385698054719,122.237627497267,-106.881824182397));
#21478=CARTESIAN_POINT('Ctrl Pts',(102.38494568036,122.237641657879,-106.882566882091));
#21479=CARTESIAN_POINT('Ctrl Pts',(102.384158609961,122.237656471514,-106.883343831673));
#21480=CARTESIAN_POINT('Ctrl Pts',(102.383368857533,122.23767247258,-106.884123555709));
#21481=CARTESIAN_POINT('Ctrl Pts',(102.382551422227,122.237690305677,-106.88493080553));
#21482=CARTESIAN_POINT('Ctrl Pts',(102.381638832476,122.237710214654,-106.885832024142));
#21483=CARTESIAN_POINT('Ctrl Pts',(102.380692303048,122.237732447118,-106.886766994239));
#21484=CARTESIAN_POINT('Ctrl Pts',(102.379730424866,122.237756826022,-106.887717360133));
#21485=CARTESIAN_POINT('Ctrl Pts',(102.378472971641,122.237788696307,-106.888959763465));
#21486=CARTESIAN_POINT('Ctrl Pts',(102.377191008879,122.237824333785,-106.890226781854));
#21487=CARTESIAN_POINT('Ctrl Pts',(102.375999399065,122.237860099073,-106.891404811914));
#21488=CARTESIAN_POINT('Ctrl Pts',(102.375025543541,122.237889328627,-106.892367569243));
#21489=CARTESIAN_POINT('Ctrl Pts',(102.374115298158,122.237918483816,-106.893267661284));
#21490=CARTESIAN_POINT('Ctrl Pts',(102.373329088986,122.237944709538,-106.894045268365));
#21491=CARTESIAN_POINT('Ctrl Pts',(102.372644486302,122.237967545954,-106.894722380657));
#21492=CARTESIAN_POINT('Ctrl Pts',(102.372054836573,122.237988087761,-106.895305724143));
#21493=CARTESIAN_POINT('Ctrl Pts',(102.371575586146,122.238005126535,-106.895779966782));
#21494=CARTESIAN_POINT('Ctrl Pts',(102.371132620484,122.238020875278,-106.896218303804));
#21495=CARTESIAN_POINT('Ctrl Pts',(102.370784467068,122.238033598544,-106.896562942416));
#21496=CARTESIAN_POINT('Ctrl Pts',(102.37051184886,122.238043654136,-106.896832907358));
#21497=CARTESIAN_POINT('Ctrl Pts',(102.370258564229,122.238052996604,-106.897083726888));
#21498=CARTESIAN_POINT('Ctrl Pts',(102.370070698614,122.238060029675,-106.897269873308));
#21499=CARTESIAN_POINT('Ctrl Pts',(102.369899836044,122.238066462969,-106.897439207673));
#21500=CARTESIAN_POINT('Ctrl Pts',(102.369866530577,122.238067716982,-106.897472215253));
#21501=CARTESIAN_POINT('Ctrl Pts',(102.369833758754,122.238068952964,-106.897504695245));
#21502=CARTESIAN_POINT('Ctrl Pts',(102.369800991998,122.238070190751,-106.897537170301));
#21503=CARTESIAN_POINT('Ctrl Pts',(102.652462829699,122.238070190751,-107.180199008002));
#21504=CARTESIAN_POINT('Ctrl Pts',(102.558242217132,122.238070190751,-107.085978395435));
#21505=CARTESIAN_POINT('Ctrl Pts',(102.464021604565,122.238070190751,-106.991757782868));
#21506=CARTESIAN_POINT('Ctrl Pts',(102.369800991998,122.238070190751,-106.897537170301));
#21507=CARTESIAN_POINT('Ctrl Pts',(102.652462829699,126.999429809249,-107.180199008002));
#21508=CARTESIAN_POINT('Ctrl Pts',(102.654130305345,126.999493365079,-107.178516554556));
#21509=CARTESIAN_POINT('Ctrl Pts',(102.666332978446,126.999932126902,-107.166174350405));
#21510=CARTESIAN_POINT('Ctrl Pts',(102.679714927635,126.999995922473,-107.152608326559));
#21511=CARTESIAN_POINT('Ctrl Pts',(102.681877591696,127.,-107.150421407138));
#21512=CARTESIAN_POINT('Ctrl Pts',(102.682294060251,127.,-107.15));
#21513=CARTESIAN_POINT('Ctrl Pts',(102.558242217132,126.999429809249,-107.085978395435));
#21514=CARTESIAN_POINT('Ctrl Pts',(102.559914685378,126.999493365079,-107.084300934589));
#21515=CARTESIAN_POINT('Ctrl Pts',(102.572170689839,126.999932126902,-107.072012061799));
#21516=CARTESIAN_POINT('Ctrl Pts',(102.585604763057,126.999995922473,-107.058498161981));
#21517=CARTESIAN_POINT('Ctrl Pts',(102.587777925418,127.,-107.05632174086));
#21518=CARTESIAN_POINT('Ctrl Pts',(102.588196040168,127.,-107.055901979916));
#21519=CARTESIAN_POINT('Ctrl Pts',(102.464021604565,126.999429809249,-106.991757782868));
#21520=CARTESIAN_POINT('Ctrl Pts',(102.465699065411,126.999493365079,-106.990085314622));
#21521=CARTESIAN_POINT('Ctrl Pts',(102.478028719002,127.000007589963,-106.97782931016));
#21522=CARTESIAN_POINT('Ctrl Pts',(102.491507491221,126.999950469076,-106.964395236943));
#21523=CARTESIAN_POINT('Ctrl Pts',(102.49367825914,127.,-106.962222074582));
#21524=CARTESIAN_POINT('Ctrl Pts',(102.494098020084,127.,-106.961803959832));
#21525=CARTESIAN_POINT('Ctrl Pts',(102.369800991998,126.999429809249,-106.897537170301));
#21526=CARTESIAN_POINT('Ctrl Pts',(102.371483445444,126.999493365079,-106.895869694655));
#21527=CARTESIAN_POINT('Ctrl Pts',(102.383825649594,126.999932126902,-106.883667021554));
#21528=CARTESIAN_POINT('Ctrl Pts',(102.397391673441,126.999995922473,-106.870285072365));
#21529=CARTESIAN_POINT('Ctrl Pts',(102.399578592862,127.,-106.868122408304));
#21530=CARTESIAN_POINT('Ctrl Pts',(102.4,127.,-106.867705939749));
#21531=CARTESIAN_POINT('',(102.369800991998,126.999429809249,-106.897537170301));
#21532=CARTESIAN_POINT('Ctrl Pts',(102.369800991998,126.999429809249,-106.897537170301));
#21533=CARTESIAN_POINT('Ctrl Pts',(102.464021604565,126.999429809249,-106.991757782868));
#21534=CARTESIAN_POINT('Ctrl Pts',(102.558242217132,126.999429809249,-107.085978395435));
#21535=CARTESIAN_POINT('Ctrl Pts',(102.652462829699,126.999429809249,-107.180199008002));
#21536=CARTESIAN_POINT('',(102.4,127.,-106.867705939749));
#21537=CARTESIAN_POINT('Ctrl Pts',(102.369800991998,126.999429809249,-106.897537170301));
#21538=CARTESIAN_POINT('Ctrl Pts',(102.369969414495,126.999436171524,-106.897370247161));
#21539=CARTESIAN_POINT('Ctrl Pts',(102.370141090614,126.999442617638,-106.897200107149));
#21540=CARTESIAN_POINT('Ctrl Pts',(102.370371942661,126.99945117313,-106.896971463311));
#21541=CARTESIAN_POINT('Ctrl Pts',(102.370626717108,126.999460615197,-106.896719125902));
#21542=CARTESIAN_POINT('Ctrl Pts',(102.370953495837,126.999472627869,-106.896395602126));
#21543=CARTESIAN_POINT('Ctrl Pts',(102.371379973835,126.999487894907,-106.895973543409));
#21544=CARTESIAN_POINT('Ctrl Pts',(102.3718562674,126.999504945239,-106.895502185326));
#21545=CARTESIAN_POINT('Ctrl Pts',(102.372456436239,126.999526020176,-106.894908400156));
#21546=CARTESIAN_POINT('Ctrl Pts',(102.373166559589,126.999549852402,-106.894206022241));
#21547=CARTESIAN_POINT('Ctrl Pts',(102.374064709175,126.999579994917,-106.893317668923));
#21548=CARTESIAN_POINT('Ctrl Pts',(102.3751373305,126.999614390365,-106.892257012151));
#21549=CARTESIAN_POINT('Ctrl Pts',(102.376288177261,126.999648516201,-106.891119331007));
#21550=CARTESIAN_POINT('Ctrl Pts',(102.37744967607,126.9996829579,-106.889971119675));
#21551=CARTESIAN_POINT('Ctrl Pts',(102.378685391777,126.999716919438,-106.888749855389));
#21552=CARTESIAN_POINT('Ctrl Pts',(102.37989486891,126.999747324912,-106.887554886453));
#21553=CARTESIAN_POINT('Ctrl Pts',(102.380800598231,126.999770094362,-106.886660021744));
#21554=CARTESIAN_POINT('Ctrl Pts',(102.381691076037,126.999790925398,-106.885780431506));
#21555=CARTESIAN_POINT('Ctrl Pts',(102.382551711391,126.999809700632,-106.884930519969));
#21556=CARTESIAN_POINT('Ctrl Pts',(102.383333112013,126.999826747316,-106.884158855871));
#21557=CARTESIAN_POINT('Ctrl Pts',(102.384089516105,126.999842123653,-106.88341204808));
#21558=CARTESIAN_POINT('Ctrl Pts',(102.384841888611,126.999856381896,-106.882669339904));
#21559=CARTESIAN_POINT('Ctrl Pts',(102.385628946577,126.999871297464,-106.881892391808));
#21560=CARTESIAN_POINT('Ctrl Pts',(102.386418854424,126.999885130105,-106.881112751621));
#21561=CARTESIAN_POINT('Ctrl Pts',(102.387236599899,126.999898178281,-106.880305665985));
#21562=CARTESIAN_POINT('Ctrl Pts',(102.388149547401,126.999912745528,-106.879404619342));
#21563=CARTESIAN_POINT('Ctrl Pts',(102.389096629821,126.999926273619,-106.878469920115));
#21564=CARTESIAN_POINT('Ctrl Pts',(102.390059211459,126.999938235568,-106.877519896475));
#21565=CARTESIAN_POINT('Ctrl Pts',(102.391317652362,126.999953874144,-106.876277873397));
#21566=CARTESIAN_POINT('Ctrl Pts',(102.39260086573,126.999966671765,-106.875011353521));
#21567=CARTESIAN_POINT('Ctrl Pts',(102.393793776563,126.999975926382,-106.873833867047));
#21568=CARTESIAN_POINT('Ctrl Pts',(102.394768572622,126.999983488862,-106.87287167512));
#21569=CARTESIAN_POINT('Ctrl Pts',(102.395679802661,126.999988722094,-106.871972161625));
#21570=CARTESIAN_POINT('Ctrl Pts',(102.396466930229,126.999992198348,-106.871195084184));
#21571=CARTESIAN_POINT('Ctrl Pts',(102.397152350636,126.999995225425,-106.870518415297));
#21572=CARTESIAN_POINT('Ctrl Pts',(102.397742760543,126.999996959481,-106.869935482459));
#21573=CARTESIAN_POINT('Ctrl Pts',(102.39822266502,126.999998025673,-106.86946159576));
#21574=CARTESIAN_POINT('Ctrl Pts',(102.398666238683,126.999999011149,-106.869023584303));
#21575=CARTESIAN_POINT('Ctrl Pts',(102.399014906889,126.999999440092,-106.868679225698));
#21576=CARTESIAN_POINT('Ctrl Pts',(102.399287955902,126.999999683121,-106.868409497879));
#21577=CARTESIAN_POINT('Ctrl Pts',(102.399541642284,126.999999908916,-106.868158897176));
#21578=CARTESIAN_POINT('Ctrl Pts',(102.399729836203,126.999999972695,-106.867972933229));
#21579=CARTESIAN_POINT('Ctrl Pts',(102.399901012219,126.999999993876,-106.867803766777));
#21580=CARTESIAN_POINT('Ctrl Pts',(102.399934365551,126.999999998003,-106.867770805005));
#21581=CARTESIAN_POINT('Ctrl Pts',(102.39996718527,127.,-106.867738369914));
#21582=CARTESIAN_POINT('Ctrl Pts',(102.4,127.,-106.867705939749));
#21583=CARTESIAN_POINT('',(102.541147030126,127.,-107.008852969874));
#21584=CARTESIAN_POINT('Ctrl Pts',(102.369800991998,126.999429809249,-106.897537170301));
#21585=CARTESIAN_POINT('Ctrl Pts',(102.172129293686,126.991962625601,-107.093449124647));
#21586=CARTESIAN_POINT('Ctrl Pts',(101.86086403162,126.852172058915,-107.425868506881));
#21587=CARTESIAN_POINT('Ctrl Pts',(101.633202511553,126.49780266677,-107.703927530503));
#21588=CARTESIAN_POINT('Ctrl Pts',(101.6,126.297687701072,-107.75));
#21589=CARTESIAN_POINT('Ctrl Pts',(101.6,126.2,-107.75));
#21590=CARTESIAN_POINT('Ctrl Pts',(102.464021604565,126.999429809249,-106.991757782868));
#21591=CARTESIAN_POINT('Ctrl Pts',(102.266936487575,126.991962625601,-107.188256318536));
#21592=CARTESIAN_POINT('Ctrl Pts',(101.94861985212,126.852172058915,-107.513624327381));
#21593=CARTESIAN_POINT('Ctrl Pts',(101.704159164201,126.49780266677,-107.774884183151));
#21594=CARTESIAN_POINT('Ctrl Pts',(101.666666666667,126.297687701072,-107.816666666667));
#21595=CARTESIAN_POINT('Ctrl Pts',(101.666666666667,126.2,-107.816666666667));
#21596=CARTESIAN_POINT('Ctrl Pts',(102.558242217132,126.999429809249,-107.085978395435));
#21597=CARTESIAN_POINT('Ctrl Pts',(102.361743681464,126.991962625601,-107.283063512425));
#21598=CARTESIAN_POINT('Ctrl Pts',(102.03637567262,126.852172058915,-107.60138014788));
#21599=CARTESIAN_POINT('Ctrl Pts',(101.775115816849,126.49780266677,-107.845840835799));
#21600=CARTESIAN_POINT('Ctrl Pts',(101.733333333333,126.297687701072,-107.883333333333));
#21601=CARTESIAN_POINT('Ctrl Pts',(101.733333333333,126.2,-107.883333333333));
#21602=CARTESIAN_POINT('Ctrl Pts',(102.652462829699,126.999429809249,-107.180199008002));
#21603=CARTESIAN_POINT('Ctrl Pts',(102.456550875353,126.991962625601,-107.377870706314));
#21604=CARTESIAN_POINT('Ctrl Pts',(102.124131493119,126.852172058915,-107.68913596838));
#21605=CARTESIAN_POINT('Ctrl Pts',(101.846072469497,126.49780266677,-107.916797488447));
#21606=CARTESIAN_POINT('Ctrl Pts',(101.8,126.297687701072,-107.95));
#21607=CARTESIAN_POINT('Ctrl Pts',(101.8,126.2,-107.95));
#21608=CARTESIAN_POINT('',(101.6,126.2,-107.75));
#21609=CARTESIAN_POINT('',(101.8,126.2,-107.95));
#21610=CARTESIAN_POINT('Ctrl Pts',(101.6,126.2,-107.75));
#21611=CARTESIAN_POINT('Ctrl Pts',(101.6,126.297687701072,-107.75));
#21612=CARTESIAN_POINT('Ctrl Pts',(101.633202511553,126.49780266677,-107.703927530503));
#21613=CARTESIAN_POINT('Ctrl Pts',(101.86086403162,126.852172058915,-107.425868506881));
#21614=CARTESIAN_POINT('Ctrl Pts',(102.172129293686,126.991962625601,-107.093449124647));
#21615=CARTESIAN_POINT('Ctrl Pts',(102.369800991998,126.999429809249,-106.897537170301));
#21616=CARTESIAN_POINT('Origin',(101.7,122.2375,-107.85));
#21617=CARTESIAN_POINT('',(101.6,123.0375,-107.75));
#21618=CARTESIAN_POINT('',(101.8,123.0375,-107.95));
#21619=CARTESIAN_POINT('',(101.6,122.2375,-107.75));
#21620=CARTESIAN_POINT('Ctrl Pts',(102.652462829699,122.238070190751,-107.180199008002));
#21621=CARTESIAN_POINT('Ctrl Pts',(102.456550875353,122.245537374399,-107.377870706314));
#21622=CARTESIAN_POINT('Ctrl Pts',(102.124131789418,122.385328018291,-107.689135810314));
#21623=CARTESIAN_POINT('Ctrl Pts',(101.84607276554,122.739697720169,-107.916797191109));
#21624=CARTESIAN_POINT('Ctrl Pts',(101.8,122.939812298928,-107.95));
#21625=CARTESIAN_POINT('Ctrl Pts',(101.8,123.0375,-107.95));
#21626=CARTESIAN_POINT('Ctrl Pts',(102.558242217132,122.238070190751,-107.085978395435));
#21627=CARTESIAN_POINT('Ctrl Pts',(102.361743681464,122.245537374399,-107.283063512425));
#21628=CARTESIAN_POINT('Ctrl Pts',(102.036375922841,122.385328018291,-107.601379943736));
#21629=CARTESIAN_POINT('Ctrl Pts',(101.775116113324,122.739697720169,-107.845840538893));
#21630=CARTESIAN_POINT('Ctrl Pts',(101.733333333333,122.939812298928,-107.883333333333));
#21631=CARTESIAN_POINT('Ctrl Pts',(101.733333333333,123.0375,-107.883333333333));
#21632=CARTESIAN_POINT('Ctrl Pts',(102.464021604565,122.238070190751,-106.991757782868));
#21633=CARTESIAN_POINT('Ctrl Pts',(102.266936487575,122.245537374399,-107.188256318536));
#21634=CARTESIAN_POINT('Ctrl Pts',(101.948620056264,122.385328018291,-107.513624077159));
#21635=CARTESIAN_POINT('Ctrl Pts',(101.704159461107,122.739697720169,-107.774883886676));
#21636=CARTESIAN_POINT('Ctrl Pts',(101.666666666667,122.939812298928,-107.816666666667));
#21637=CARTESIAN_POINT('Ctrl Pts',(101.666666666667,123.0375,-107.816666666667));
#21638=CARTESIAN_POINT('Ctrl Pts',(102.369800991998,122.238070190751,-106.897537170301));
#21639=CARTESIAN_POINT('Ctrl Pts',(102.172129293686,122.245537374399,-107.093449124647));
#21640=CARTESIAN_POINT('Ctrl Pts',(101.860864189686,122.385328018291,-107.425868210582));
#21641=CARTESIAN_POINT('Ctrl Pts',(101.633202808891,122.739697720169,-107.70392723446));
#21642=CARTESIAN_POINT('Ctrl Pts',(101.6,122.939812298928,-107.75));
#21643=CARTESIAN_POINT('Ctrl Pts',(101.6,123.0375,-107.75));
#21644=CARTESIAN_POINT('Ctrl Pts',(102.369800991998,122.238070190751,-106.897537170301));
#21645=CARTESIAN_POINT('Ctrl Pts',(102.172129293686,122.245537374399,-107.093449124647));
#21646=CARTESIAN_POINT('Ctrl Pts',(101.860864189686,122.385328018291,-107.425868210582));
#21647=CARTESIAN_POINT('Ctrl Pts',(101.633202808891,122.739697720169,-107.70392723446));
#21648=CARTESIAN_POINT('Ctrl Pts',(101.6,122.939812298928,-107.75));
#21649=CARTESIAN_POINT('Ctrl Pts',(101.6,123.0375,-107.75));
#21650=CARTESIAN_POINT('Ctrl Pts',(102.652462829699,122.238070190751,43.6801990080023));
#21651=CARTESIAN_POINT('Ctrl Pts',(102.654130305345,122.238006634921,43.678516554556));
#21652=CARTESIAN_POINT('Ctrl Pts',(102.666334669584,122.237567840162,43.6661726500475));
#21653=CARTESIAN_POINT('Ctrl Pts',(102.679715367383,122.237504071867,43.6526078837211));
#21654=CARTESIAN_POINT('Ctrl Pts',(102.681877591696,122.2375,43.6504214071384));
#21655=CARTESIAN_POINT('Ctrl Pts',(102.682294060251,122.2375,43.65));
#21656=CARTESIAN_POINT('Ctrl Pts',(102.558242217132,122.238070190751,43.5859783954351));
#21657=CARTESIAN_POINT('Ctrl Pts',(102.559914685378,122.238006634921,43.584300934589));
#21658=CARTESIAN_POINT('Ctrl Pts',(102.572172380978,122.237567840162,43.5720103614411));
#21659=CARTESIAN_POINT('Ctrl Pts',(102.585605202805,122.237504071867,43.5584977191432));
#21660=CARTESIAN_POINT('Ctrl Pts',(102.587777925418,122.2375,43.5563217408604));
#21661=CARTESIAN_POINT('Ctrl Pts',(102.588196040168,122.2375,43.5559019799162));
#21662=CARTESIAN_POINT('Ctrl Pts',(102.464021604565,122.238070190751,43.4917577828678));
#21663=CARTESIAN_POINT('Ctrl Pts',(102.465699065411,122.238006634921,43.490085314622));
#21664=CARTESIAN_POINT('Ctrl Pts',(102.478030427135,122.237492576792,43.4778276190222));
#21665=CARTESIAN_POINT('Ctrl Pts',(102.491507935396,122.237549577289,43.4643947971951));
#21666=CARTESIAN_POINT('Ctrl Pts',(102.49367825914,122.2375,43.4622220745823));
#21667=CARTESIAN_POINT('Ctrl Pts',(102.494098020084,122.2375,43.4618039598323));
#21668=CARTESIAN_POINT('Ctrl Pts',(102.369800991998,122.238070190751,43.3975371703006));
#21669=CARTESIAN_POINT('Ctrl Pts',(102.371483445444,122.238006634921,43.3958696946549));
#21670=CARTESIAN_POINT('Ctrl Pts',(102.383827349952,122.237567840162,43.3836653304159));
#21671=CARTESIAN_POINT('Ctrl Pts',(102.397392116279,122.237504071867,43.3702846326172));
#21672=CARTESIAN_POINT('Ctrl Pts',(102.399578592862,122.2375,43.3681224083043));
#21673=CARTESIAN_POINT('Ctrl Pts',(102.4,122.2375,43.3677059397485));
#21674=CARTESIAN_POINT('',(102.652462829699,122.238070190751,43.6801990080023));
#21675=CARTESIAN_POINT('Ctrl Pts',(102.682294060251,122.2375,43.65));
#21676=CARTESIAN_POINT('Ctrl Pts',(102.682127301195,122.2375,43.650168736525));
#21677=CARTESIAN_POINT('Ctrl Pts',(102.681957327238,122.237500039141,43.6503407294752));
#21678=CARTESIAN_POINT('Ctrl Pts',(102.681728880148,122.237500204467,43.6505719684178));
#21679=CARTESIAN_POINT('Ctrl Pts',(102.681476760615,122.237500386926,43.6508271691041));
#21680=CARTESIAN_POINT('Ctrl Pts',(102.681153492515,122.23750071898,43.6511544591101));
#21681=CARTESIAN_POINT('Ctrl Pts',(102.680731737107,122.237501563317,43.6515815512717));
#21682=CARTESIAN_POINT('Ctrl Pts',(102.680260720798,122.237502506272,43.6520585276647));
#21683=CARTESIAN_POINT('Ctrl Pts',(102.679667338179,122.237504104656,43.6526595049514));
#21684=CARTESIAN_POINT('Ctrl Pts',(102.678965403787,122.237507100231,43.6533705073352));
#21685=CARTESIAN_POINT('Ctrl Pts',(102.678077643409,122.237510888837,43.654269736312));
#21686=CARTESIAN_POINT('Ctrl Pts',(102.67701765694,122.237517016609,43.6553435322326));
#21687=CARTESIAN_POINT('Ctrl Pts',(102.675880626364,122.237526369906,43.6564954718404));
#21688=CARTESIAN_POINT('Ctrl Pts',(102.674732975653,122.237535810566,43.657658170837));
#21689=CARTESIAN_POINT('Ctrl Pts',(102.673512235913,122.237548536479,43.6588950097936));
#21690=CARTESIAN_POINT('Ctrl Pts',(102.672317676586,122.237563826519,43.6601053627627));
#21691=CARTESIAN_POINT('Ctrl Pts',(102.671423130776,122.237575276466,43.6610117356424));
#21692=CARTESIAN_POINT('Ctrl Pts',(102.670543794254,122.237588088159,43.6619027203553));
#21693=CARTESIAN_POINT('Ctrl Pts',(102.669694048351,122.237601826337,43.6627636895375));
#21694=CARTESIAN_POINT('Ctrl Pts',(102.66892254147,122.237614299594,43.6635453863333));
#21695=CARTESIAN_POINT('Ctrl Pts',(102.668175817601,122.237627497267,43.6643019452827));
#21696=CARTESIAN_POINT('Ctrl Pts',(102.667433117906,122.237641657879,43.665054319643));
#21697=CARTESIAN_POINT('Ctrl Pts',(102.666656168324,122.237656471514,43.6658413900421));
#21698=CARTESIAN_POINT('Ctrl Pts',(102.665876444288,122.23767247258,43.6666311424699));
#21699=CARTESIAN_POINT('Ctrl Pts',(102.665069194467,122.237690305677,43.6674485777763));
#21700=CARTESIAN_POINT('Ctrl Pts',(102.664167975855,122.237710214654,43.6683611675272));
#21701=CARTESIAN_POINT('Ctrl Pts',(102.663233005757,122.237732447118,43.6693076969552));
#21702=CARTESIAN_POINT('Ctrl Pts',(102.662282639863,122.237756826022,43.6702695751378));
#21703=CARTESIAN_POINT('Ctrl Pts',(102.661040236531,122.237788696307,43.6715270283636));
#21704=CARTESIAN_POINT('Ctrl Pts',(102.659773218141,122.237824333785,43.6728089911263));
#21705=CARTESIAN_POINT('Ctrl Pts',(102.65859518808,122.237860099073,43.6740006009409));
#21706=CARTESIAN_POINT('Ctrl Pts',(102.657632430752,122.237889328627,43.6749744564645));
#21707=CARTESIAN_POINT('Ctrl Pts',(102.656732338711,122.237918483816,43.6758847018465));
#21708=CARTESIAN_POINT('Ctrl Pts',(102.655954731631,122.237944709538,43.6766709110183));
#21709=CARTESIAN_POINT('Ctrl Pts',(102.65527761934,122.237967545954,43.6773555137014));
#21710=CARTESIAN_POINT('Ctrl Pts',(102.654694275854,122.237988087761,43.6779451634301));
#21711=CARTESIAN_POINT('Ctrl Pts',(102.654220033215,122.238005126535,43.6784244138562));
#21712=CARTESIAN_POINT('Ctrl Pts',(102.653781696193,122.238020875278,43.6788673795183));
#21713=CARTESIAN_POINT('Ctrl Pts',(102.653437057583,122.238033598544,43.6792155329338));
#21714=CARTESIAN_POINT('Ctrl Pts',(102.65316709264,122.238043654136,43.6794881511416));
#21715=CARTESIAN_POINT('Ctrl Pts',(102.65291627311,122.238052996604,43.6797414357727));
#21716=CARTESIAN_POINT('Ctrl Pts',(102.652730126691,122.238060029675,43.679929301387));
#21717=CARTESIAN_POINT('Ctrl Pts',(102.652560792326,122.238066462969,43.6801001639574));
#21718=CARTESIAN_POINT('Ctrl Pts',(102.652527784746,122.238067716982,43.6801334694235));
#21719=CARTESIAN_POINT('Ctrl Pts',(102.652495304755,122.238068952964,43.6801662412459));
#21720=CARTESIAN_POINT('Ctrl Pts',(102.652462829699,122.238070190751,43.6801990080023));
#21721=CARTESIAN_POINT('',(102.369800991998,122.238070190751,43.3975371703006));
#21722=CARTESIAN_POINT('Ctrl Pts',(102.369800991998,122.238070190751,43.3975371703006));
#21723=CARTESIAN_POINT('Ctrl Pts',(102.464021604565,122.238070190751,43.4917577828678));
#21724=CARTESIAN_POINT('Ctrl Pts',(102.558242217132,122.238070190751,43.5859783954351));
#21725=CARTESIAN_POINT('Ctrl Pts',(102.652462829699,122.238070190751,43.6801990080023));
#21726=CARTESIAN_POINT('Ctrl Pts',(102.369800991998,122.238070190751,43.3975371703006));
#21727=CARTESIAN_POINT('Ctrl Pts',(102.369969414495,122.238063828476,43.3973702471606));
#21728=CARTESIAN_POINT('Ctrl Pts',(102.370141090614,122.238057382362,43.397200107149));
#21729=CARTESIAN_POINT('Ctrl Pts',(102.370371942661,122.23804882687,43.3969714633111));
#21730=CARTESIAN_POINT('Ctrl Pts',(102.370626717108,122.238039384803,43.3967191259023));
#21731=CARTESIAN_POINT('Ctrl Pts',(102.370953495837,122.238027372131,43.3963956021262));
#21732=CARTESIAN_POINT('Ctrl Pts',(102.371379973835,122.238012105093,43.3959735434091));
#21733=CARTESIAN_POINT('Ctrl Pts',(102.3718562674,122.237995054761,43.3955021853265));
#21734=CARTESIAN_POINT('Ctrl Pts',(102.372456436239,122.237973979824,43.3949084001559));
#21735=CARTESIAN_POINT('Ctrl Pts',(102.373166559589,122.237950147598,43.3942060222409));
#21736=CARTESIAN_POINT('Ctrl Pts',(102.374064709175,122.237920005083,43.3933176689235));
#21737=CARTESIAN_POINT('Ctrl Pts',(102.3751373305,122.237885609635,43.3922570121515));
#21738=CARTESIAN_POINT('Ctrl Pts',(102.376288177261,122.237851483799,43.391119331008));
#21739=CARTESIAN_POINT('Ctrl Pts',(102.37744967607,122.2378170421,43.3899711196755));
#21740=CARTESIAN_POINT('Ctrl Pts',(102.378685391777,122.237783080562,43.3887498553894));
#21741=CARTESIAN_POINT('Ctrl Pts',(102.37989486891,122.237752675088,43.3875548864534));
#21742=CARTESIAN_POINT('Ctrl Pts',(102.38080059823,122.237729905638,43.386660021744));
#21743=CARTESIAN_POINT('Ctrl Pts',(102.381691076037,122.237709074602,43.385780431506));
#21744=CARTESIAN_POINT('Ctrl Pts',(102.38255171139,122.237690299368,43.3849305199691));
#21745=CARTESIAN_POINT('Ctrl Pts',(102.383333112017,122.237673252684,43.3841588558664));
#21746=CARTESIAN_POINT('Ctrl Pts',(102.384089516114,122.237657876347,43.3834120480707));
#21747=CARTESIAN_POINT('Ctrl Pts',(102.384841888625,122.237643618104,43.3826693398905));
#21748=CARTESIAN_POINT('Ctrl Pts',(102.385628946591,122.237628702536,43.3818923917941));
#21749=CARTESIAN_POINT('Ctrl Pts',(102.386418854439,122.237614869895,43.3811127516064));
#21750=CARTESIAN_POINT('Ctrl Pts',(102.387236599914,122.237601821718,43.3803056659701));
#21751=CARTESIAN_POINT('Ctrl Pts',(102.388149547418,122.237587254471,43.3794046193259));
#21752=CARTESIAN_POINT('Ctrl Pts',(102.389096629839,122.237573726381,43.3784699200974));
#21753=CARTESIAN_POINT('Ctrl Pts',(102.390059211478,122.237561764432,43.3775198964558));
#21754=CARTESIAN_POINT('Ctrl Pts',(102.391317652386,122.237546125856,43.3762778733733));
#21755=CARTESIAN_POINT('Ctrl Pts',(102.392600865758,122.237533328235,43.3750113534931));
#21756=CARTESIAN_POINT('Ctrl Pts',(102.393793776595,122.237524073618,43.3738338670164));
#21757=CARTESIAN_POINT('Ctrl Pts',(102.394768572651,122.237516511138,43.372871675092));
#21758=CARTESIAN_POINT('Ctrl Pts',(102.395679802686,122.237511277906,43.371972161601));
#21759=CARTESIAN_POINT('Ctrl Pts',(102.39646693025,122.237507801652,43.3711950841639));
#21760=CARTESIAN_POINT('Ctrl Pts',(102.397152350654,122.237504774575,43.3705184152794));
#21761=CARTESIAN_POINT('Ctrl Pts',(102.397742760559,122.237503040519,43.3699354824433));
#21762=CARTESIAN_POINT('Ctrl Pts',(102.398222665033,122.237501974327,43.3694615957471));
#21763=CARTESIAN_POINT('Ctrl Pts',(102.398666238694,122.237500988851,43.3690235842925));
#21764=CARTESIAN_POINT('Ctrl Pts',(102.399014906898,122.237500559908,43.3686792256888));
#21765=CARTESIAN_POINT('Ctrl Pts',(102.399287955909,122.237500316879,43.368409497871));
#21766=CARTESIAN_POINT('Ctrl Pts',(102.39954164229,122.237500091084,43.3681588971694));
#21767=CARTESIAN_POINT('Ctrl Pts',(102.399729836208,122.237500027304,43.3679729332236));
#21768=CARTESIAN_POINT('Ctrl Pts',(102.399901012224,122.237500006124,43.3678037667716));
#21769=CARTESIAN_POINT('Ctrl Pts',(102.399934365554,122.237500001997,43.3677708050016));
#21770=CARTESIAN_POINT('Ctrl Pts',(102.399967185272,122.2375,43.3677383699122));
#21771=CARTESIAN_POINT('Ctrl Pts',(102.4,122.2375,43.3677059397485));
#21772=CARTESIAN_POINT('Ctrl Pts',(102.369800991998,126.999429809249,43.3975371703006));
#21773=CARTESIAN_POINT('Ctrl Pts',(102.371483445444,126.999493365079,43.395869694655));
#21774=CARTESIAN_POINT('Ctrl Pts',(102.383827204795,126.999932157025,43.3836654747861));
#21775=CARTESIAN_POINT('Ctrl Pts',(102.397392078533,126.999995927652,43.3702846700996));
#21776=CARTESIAN_POINT('Ctrl Pts',(102.399578592862,127.,43.3681224083043));
#21777=CARTESIAN_POINT('Ctrl Pts',(102.4,127.,43.3677059397485));
#21778=CARTESIAN_POINT('Ctrl Pts',(102.464021604565,126.999429809249,43.4917577828679));
#21779=CARTESIAN_POINT('Ctrl Pts',(102.465699065411,126.999493365079,43.490085314622));
#21780=CARTESIAN_POINT('Ctrl Pts',(102.477989493402,126.999932157025,43.4778277633925));
#21781=CARTESIAN_POINT('Ctrl Pts',(102.491502243111,126.999995927652,43.4643948346774));
#21782=CARTESIAN_POINT('Ctrl Pts',(102.49367825914,127.,43.4622220745824));
#21783=CARTESIAN_POINT('Ctrl Pts',(102.494098020084,127.,43.4618039598323));
#21784=CARTESIAN_POINT('Ctrl Pts',(102.558242217132,126.999429809249,43.5859783954351));
#21785=CARTESIAN_POINT('Ctrl Pts',(102.559914685378,126.999493365079,43.584300934589));
#21786=CARTESIAN_POINT('Ctrl Pts',(102.572172236607,127.000007437442,43.5719697186859));
#21787=CARTESIAN_POINT('Ctrl Pts',(102.585605165322,126.999950426665,43.558492102464));
#21788=CARTESIAN_POINT('Ctrl Pts',(102.587777925418,127.,43.5563217408604));
#21789=CARTESIAN_POINT('Ctrl Pts',(102.588196040168,127.,43.5559019799162));
#21790=CARTESIAN_POINT('Ctrl Pts',(102.652462829699,126.999429809249,43.6801990080024));
#21791=CARTESIAN_POINT('Ctrl Pts',(102.654130305345,126.999493365079,43.6785165545561));
#21792=CARTESIAN_POINT('Ctrl Pts',(102.666334525214,126.999932157025,43.6661727952046));
#21793=CARTESIAN_POINT('Ctrl Pts',(102.6797153299,126.999995927652,43.6526079214671));
#21794=CARTESIAN_POINT('Ctrl Pts',(102.681877591696,127.,43.6504214071384));
#21795=CARTESIAN_POINT('Ctrl Pts',(102.682294060251,127.,43.65));
#21796=CARTESIAN_POINT('',(102.4,127.,43.3677059397485));
#21797=CARTESIAN_POINT('',(102.369800991998,126.999429809249,43.3975371703006));
#21798=CARTESIAN_POINT('Ctrl Pts',(102.4,127.,43.3677059397485));
#21799=CARTESIAN_POINT('Ctrl Pts',(102.399831263475,127.,43.3678726988052));
#21800=CARTESIAN_POINT('Ctrl Pts',(102.399659270525,126.999999960859,43.3680426727623));
#21801=CARTESIAN_POINT('Ctrl Pts',(102.399428031582,126.999999795533,43.3682711198523));
#21802=CARTESIAN_POINT('Ctrl Pts',(102.399172830896,126.999999613074,43.368523239385));
#21803=CARTESIAN_POINT('Ctrl Pts',(102.39884554089,126.99999928102,43.3688465074853));
#21804=CARTESIAN_POINT('Ctrl Pts',(102.398418448728,126.999998436683,43.3692682628935));
#21805=CARTESIAN_POINT('Ctrl Pts',(102.397941472335,126.999997493728,43.3697392792018));
#21806=CARTESIAN_POINT('Ctrl Pts',(102.397340495048,126.999995895344,43.3703326618209));
#21807=CARTESIAN_POINT('Ctrl Pts',(102.396629492664,126.999992899769,43.3710345962131));
#21808=CARTESIAN_POINT('Ctrl Pts',(102.395730263688,126.999989111163,43.3719223565914));
#21809=CARTESIAN_POINT('Ctrl Pts',(102.394656467767,126.999982983391,43.3729823430605));
#21810=CARTESIAN_POINT('Ctrl Pts',(102.393504528159,126.999973630094,43.3741193736366));
#21811=CARTESIAN_POINT('Ctrl Pts',(102.392341829162,126.999964189434,43.3752670243476));
#21812=CARTESIAN_POINT('Ctrl Pts',(102.391104990206,126.999951463521,43.3764877640872));
#21813=CARTESIAN_POINT('Ctrl Pts',(102.389894637237,126.999936173481,43.3776823234144));
#21814=CARTESIAN_POINT('Ctrl Pts',(102.388988264357,126.999924723534,43.3785768692246));
#21815=CARTESIAN_POINT('Ctrl Pts',(102.388097279644,126.999911911841,43.379456205747));
#21816=CARTESIAN_POINT('Ctrl Pts',(102.387236310462,126.999898173663,43.3803059516493));
#21817=CARTESIAN_POINT('Ctrl Pts',(102.386454613667,126.999885700406,43.3810774585302));
#21818=CARTESIAN_POINT('Ctrl Pts',(102.385698054718,126.999872502733,43.3818241823982));
#21819=CARTESIAN_POINT('Ctrl Pts',(102.384945680359,126.999858342121,43.3825668820919));
#21820=CARTESIAN_POINT('Ctrl Pts',(102.38415860996,126.999843528486,43.3833438316742));
#21821=CARTESIAN_POINT('Ctrl Pts',(102.383368857532,126.99982752742,43.3841235557102));
#21822=CARTESIAN_POINT('Ctrl Pts',(102.382551422226,126.999809694323,43.3849308055307));
#21823=CARTESIAN_POINT('Ctrl Pts',(102.381638832475,126.999789785346,43.3858320241431));
#21824=CARTESIAN_POINT('Ctrl Pts',(102.380692303047,126.999767552882,43.3867669942407));
#21825=CARTESIAN_POINT('Ctrl Pts',(102.379730424864,126.999743173978,43.3877173601347));
#21826=CARTESIAN_POINT('Ctrl Pts',(102.378472971639,126.999711303693,43.3889597634663));
#21827=CARTESIAN_POINT('Ctrl Pts',(102.377191008877,126.999675666215,43.390226781856));
#21828=CARTESIAN_POINT('Ctrl Pts',(102.375999399063,126.999639900927,43.3914048119161));
#21829=CARTESIAN_POINT('Ctrl Pts',(102.375025543539,126.999610671373,43.3923675692448));
#21830=CARTESIAN_POINT('Ctrl Pts',(102.374115298156,126.999581516184,43.3932676612859));
#21831=CARTESIAN_POINT('Ctrl Pts',(102.373329088984,126.999555290462,43.3940452683668));
#21832=CARTESIAN_POINT('Ctrl Pts',(102.372644486301,126.999532454046,43.3947223806583));
#21833=CARTESIAN_POINT('Ctrl Pts',(102.372054836572,126.999511912239,43.3953057241444));
#21834=CARTESIAN_POINT('Ctrl Pts',(102.371575586145,126.999494873465,43.3957799667835));
#21835=CARTESIAN_POINT('Ctrl Pts',(102.371132620483,126.999479124722,43.3962183038054));
#21836=CARTESIAN_POINT('Ctrl Pts',(102.370784467067,126.999466401456,43.3965629424164));
#21837=CARTESIAN_POINT('Ctrl Pts',(102.370511848859,126.999456345864,43.3968329073587));
#21838=CARTESIAN_POINT('Ctrl Pts',(102.370258564228,126.999447003396,43.3970837268889));
#21839=CARTESIAN_POINT('Ctrl Pts',(102.370070698614,126.999439970325,43.3972698733084));
#21840=CARTESIAN_POINT('Ctrl Pts',(102.369899836043,126.999433537031,43.3974392076734));
#21841=CARTESIAN_POINT('Ctrl Pts',(102.369866530577,126.999432283018,43.3974722152535));
#21842=CARTESIAN_POINT('Ctrl Pts',(102.369833758754,126.999431047036,43.3975046952453));
#21843=CARTESIAN_POINT('Ctrl Pts',(102.369800991998,126.999429809249,43.3975371703006));
#21844=CARTESIAN_POINT('',(102.652462829699,126.999429809249,43.6801990080024));
#21845=CARTESIAN_POINT('Ctrl Pts',(102.652462829699,126.999429809249,43.6801990080024));
#21846=CARTESIAN_POINT('Ctrl Pts',(102.558242217132,126.999429809249,43.5859783954351));
#21847=CARTESIAN_POINT('Ctrl Pts',(102.464021604565,126.999429809249,43.4917577828679));
#21848=CARTESIAN_POINT('Ctrl Pts',(102.369800991998,126.999429809249,43.3975371703006));
#21849=CARTESIAN_POINT('',(102.682294060251,127.,43.65));
#21850=CARTESIAN_POINT('Ctrl Pts',(102.652462829699,126.999429809249,43.6801990080024));
#21851=CARTESIAN_POINT('Ctrl Pts',(102.652629752839,126.999436171524,43.6800305855052));
#21852=CARTESIAN_POINT('Ctrl Pts',(102.652799892851,126.999442617638,43.6798589093858));
#21853=CARTESIAN_POINT('Ctrl Pts',(102.653028536689,126.99945117313,43.6796280573389));
#21854=CARTESIAN_POINT('Ctrl Pts',(102.653280874098,126.999460615197,43.6793732828919));
#21855=CARTESIAN_POINT('Ctrl Pts',(102.653604397874,126.999472627869,43.6790465041629));
#21856=CARTESIAN_POINT('Ctrl Pts',(102.654026456591,126.999487894907,43.6786200261654));
#21857=CARTESIAN_POINT('Ctrl Pts',(102.654497814673,126.999504945239,43.6781437326003));
#21858=CARTESIAN_POINT('Ctrl Pts',(102.655091599844,126.999526020176,43.6775435637606));
#21859=CARTESIAN_POINT('Ctrl Pts',(102.655793977759,126.999549852402,43.6768334404111));
#21860=CARTESIAN_POINT('Ctrl Pts',(102.656682331077,126.999579994917,43.6759352908252));
#21861=CARTESIAN_POINT('Ctrl Pts',(102.657742987849,126.999614390365,43.6748626694998));
#21862=CARTESIAN_POINT('Ctrl Pts',(102.658880668993,126.999648516201,43.6737118227386));
#21863=CARTESIAN_POINT('Ctrl Pts',(102.660028880325,126.9996829579,43.6725503239297));
#21864=CARTESIAN_POINT('Ctrl Pts',(102.661250144611,126.999716919438,43.6713146082226));
#21865=CARTESIAN_POINT('Ctrl Pts',(102.662445113547,126.999747324912,43.67010513109));
#21866=CARTESIAN_POINT('Ctrl Pts',(102.663339978256,126.999770094362,43.6691994017692));
#21867=CARTESIAN_POINT('Ctrl Pts',(102.664219568494,126.999790925398,43.6683089239629));
#21868=CARTESIAN_POINT('Ctrl Pts',(102.665069480031,126.999809700632,43.6674482886094));
#21869=CARTESIAN_POINT('Ctrl Pts',(102.66584114413,126.999826747316,43.6666668879864));
#21870=CARTESIAN_POINT('Ctrl Pts',(102.666587951922,126.999842123653,43.6659104838931));
#21871=CARTESIAN_POINT('Ctrl Pts',(102.667330660098,126.999856381896,43.6651581113864));
#21872=CARTESIAN_POINT('Ctrl Pts',(102.668107608194,126.999871297464,43.6643710534204));
#21873=CARTESIAN_POINT('Ctrl Pts',(102.668887248382,126.999885130105,43.6635811455735));
#21874=CARTESIAN_POINT('Ctrl Pts',(102.669694334017,126.999898178281,43.6627634000984));
#21875=CARTESIAN_POINT('Ctrl Pts',(102.670595380661,126.999912745528,43.6618504525959));
#21876=CARTESIAN_POINT('Ctrl Pts',(102.671530079888,126.999926273619,43.6609033701756));
#21877=CARTESIAN_POINT('Ctrl Pts',(102.672480103529,126.999938235568,43.6599407885377));
#21878=CARTESIAN_POINT('Ctrl Pts',(102.673722126608,126.999953874144,43.6586823476335));
#21879=CARTESIAN_POINT('Ctrl Pts',(102.674988646484,126.999966671765,43.6573991342643));
#21880=CARTESIAN_POINT('Ctrl Pts',(102.676166132959,126.999975926382,43.6562062234303));
#21881=CARTESIAN_POINT('Ctrl Pts',(102.677128324886,126.999983488862,43.6552314273719));
#21882=CARTESIAN_POINT('Ctrl Pts',(102.67802783838,126.999988722094,43.6543201973338));
#21883=CARTESIAN_POINT('Ctrl Pts',(102.67880491582,126.999992198348,43.6535330697665));
#21884=CARTESIAN_POINT('Ctrl Pts',(102.679481584706,126.999995225425,43.6528476493604));
#21885=CARTESIAN_POINT('Ctrl Pts',(102.680064517544,126.999996959481,43.6522572394536));
#21886=CARTESIAN_POINT('Ctrl Pts',(102.680538404243,126.999998025673,43.6517773349774));
#21887=CARTESIAN_POINT('Ctrl Pts',(102.680976415699,126.999999011149,43.6513337613144));
#21888=CARTESIAN_POINT('Ctrl Pts',(102.681320774304,126.999999440092,43.6509850931095));
#21889=CARTESIAN_POINT('Ctrl Pts',(102.681590502123,126.999999683121,43.6507120440968));
#21890=CARTESIAN_POINT('Ctrl Pts',(102.681841102826,126.999999908916,43.650458357715));
#21891=CARTESIAN_POINT('Ctrl Pts',(102.682027066772,126.999999972695,43.6502701637959));
#21892=CARTESIAN_POINT('Ctrl Pts',(102.682196233224,126.999999993876,43.6500989877796));
#21893=CARTESIAN_POINT('Ctrl Pts',(102.682229194996,126.999999998003,43.6500656344483));
#21894=CARTESIAN_POINT('Ctrl Pts',(102.682261630086,127.,43.6500328147295));
#21895=CARTESIAN_POINT('Ctrl Pts',(102.682294060251,127.,43.65));
#21896=CARTESIAN_POINT('',(102.541147030126,127.,43.5088529698743));
#21897=CARTESIAN_POINT('Ctrl Pts',(102.652462829699,126.999429809249,43.6801990080024));
#21898=CARTESIAN_POINT('Ctrl Pts',(102.456550875353,126.991962625601,43.8778707063143));
#21899=CARTESIAN_POINT('Ctrl Pts',(102.124136995242,126.852170699062,44.1891330663933));
#21900=CARTESIAN_POINT('Ctrl Pts',(101.846077990743,126.497795401137,44.4167919209351));
#21901=CARTESIAN_POINT('Ctrl Pts',(101.8,126.297687701072,44.45));
#21902=CARTESIAN_POINT('Ctrl Pts',(101.8,126.2,44.45));
#21903=CARTESIAN_POINT('Ctrl Pts',(102.558242217132,126.999429809249,43.5859783954351));
#21904=CARTESIAN_POINT('Ctrl Pts',(102.361743681464,126.991962625601,43.7830635124252));
#21905=CARTESIAN_POINT('Ctrl Pts',(102.03638030803,126.852170699062,44.1013763791816));
#21906=CARTESIAN_POINT('Ctrl Pts',(101.775121353517,126.497795401137,44.3458352837092));
#21907=CARTESIAN_POINT('Ctrl Pts',(101.733333333333,126.297687701072,44.3833333333333));
#21908=CARTESIAN_POINT('Ctrl Pts',(101.733333333333,126.2,44.3833333333333));
#21909=CARTESIAN_POINT('Ctrl Pts',(102.464021604565,126.999429809249,43.4917577828679));
#21910=CARTESIAN_POINT('Ctrl Pts',(102.266936487575,126.991962625601,43.6882563185361));
#21911=CARTESIAN_POINT('Ctrl Pts',(101.948623620818,126.852170699062,44.0136196919698));
#21912=CARTESIAN_POINT('Ctrl Pts',(101.704164716291,126.497795401137,44.2748786464833));
#21913=CARTESIAN_POINT('Ctrl Pts',(101.666666666667,126.297687701072,44.3166666666667));
#21914=CARTESIAN_POINT('Ctrl Pts',(101.666666666667,126.2,44.3166666666667));
#21915=CARTESIAN_POINT('Ctrl Pts',(102.369800991998,126.999429809249,43.3975371703006));
#21916=CARTESIAN_POINT('Ctrl Pts',(102.172129293686,126.991962625601,43.5934491246469));
#21917=CARTESIAN_POINT('Ctrl Pts',(101.860866933607,126.852170699062,43.9258630047581));
#21918=CARTESIAN_POINT('Ctrl Pts',(101.633208079065,126.497795401137,44.2039220092575));
#21919=CARTESIAN_POINT('Ctrl Pts',(101.6,126.297687701072,44.25));
#21920=CARTESIAN_POINT('Ctrl Pts',(101.6,126.2,44.25));
#21921=CARTESIAN_POINT('',(101.6,126.2,44.25));
#21922=CARTESIAN_POINT('Ctrl Pts',(102.369800991998,126.999429809249,43.3975371703006));
#21923=CARTESIAN_POINT('Ctrl Pts',(102.172129293686,126.991962625601,43.5934491246469));
#21924=CARTESIAN_POINT('Ctrl Pts',(101.860866933607,126.852170699062,43.9258630047581));
#21925=CARTESIAN_POINT('Ctrl Pts',(101.633208079065,126.497795401137,44.2039220092575));
#21926=CARTESIAN_POINT('Ctrl Pts',(101.6,126.297687701072,44.25));
#21927=CARTESIAN_POINT('Ctrl Pts',(101.6,126.2,44.25));
#21928=CARTESIAN_POINT('',(101.8,126.2,44.45));
#21929=CARTESIAN_POINT('',(101.6,126.2,44.25));
#21930=CARTESIAN_POINT('Ctrl Pts',(101.8,126.2,44.45));
#21931=CARTESIAN_POINT('Ctrl Pts',(101.8,126.297687701072,44.45));
#21932=CARTESIAN_POINT('Ctrl Pts',(101.846077990743,126.497795401137,44.4167919209351));
#21933=CARTESIAN_POINT('Ctrl Pts',(102.124136995242,126.852170699062,44.1891330663933));
#21934=CARTESIAN_POINT('Ctrl Pts',(102.456550875353,126.991962625601,43.8778707063143));
#21935=CARTESIAN_POINT('Ctrl Pts',(102.652462829699,126.999429809249,43.6801990080024));
#21936=CARTESIAN_POINT('Origin',(101.7,122.2375,44.35));
#21937=CARTESIAN_POINT('',(101.6,123.0375,44.25));
#21938=CARTESIAN_POINT('',(101.6,122.2375,44.25));
#21939=CARTESIAN_POINT('',(101.8,123.0375,44.45));
#21940=CARTESIAN_POINT('',(101.6,123.0375,44.25));
#21941=CARTESIAN_POINT('',(101.8,122.2375,44.45));
#21942=CARTESIAN_POINT('Ctrl Pts',(101.8,123.0375,44.45));
#21943=CARTESIAN_POINT('Ctrl Pts',(101.8,122.939812298928,44.45));
#21944=CARTESIAN_POINT('Ctrl Pts',(101.846078418479,122.739705166155,44.4167914876269));
#21945=CARTESIAN_POINT('Ctrl Pts',(102.124137419351,122.385329399097,44.1891328457024));
#21946=CARTESIAN_POINT('Ctrl Pts',(102.456550875353,122.245537374399,43.8778707063143));
#21947=CARTESIAN_POINT('Ctrl Pts',(102.652462829699,122.238070190751,43.6801990080023));
#21948=CARTESIAN_POINT('Ctrl Pts',(101.733333333333,123.0375,44.3833333333333));
#21949=CARTESIAN_POINT('Ctrl Pts',(101.733333333333,122.939812298928,44.3833333333333));
#21950=CARTESIAN_POINT('Ctrl Pts',(101.77512178311,122.739705166155,44.3458348522582));
#21951=CARTESIAN_POINT('Ctrl Pts',(102.036380664333,122.385329399097,44.1013760906846));
#21952=CARTESIAN_POINT('Ctrl Pts',(102.361743681464,122.245537374399,43.7830635124252));
#21953=CARTESIAN_POINT('Ctrl Pts',(102.558242217132,122.238070190751,43.5859783954351));
#21954=CARTESIAN_POINT('Ctrl Pts',(101.666666666667,123.0375,44.3166666666667));
#21955=CARTESIAN_POINT('Ctrl Pts',(101.666666666667,122.939812298928,44.3166666666667));
#21956=CARTESIAN_POINT('Ctrl Pts',(101.704165147742,122.739705166155,44.2748782168895));
#21957=CARTESIAN_POINT('Ctrl Pts',(101.948623909315,122.385329399097,44.0136193356668));
#21958=CARTESIAN_POINT('Ctrl Pts',(102.266936487575,122.245537374399,43.688256318536));
#21959=CARTESIAN_POINT('Ctrl Pts',(102.464021604565,122.238070190751,43.4917577828678));
#21960=CARTESIAN_POINT('Ctrl Pts',(101.6,123.0375,44.25));
#21961=CARTESIAN_POINT('Ctrl Pts',(101.6,122.939812298928,44.25));
#21962=CARTESIAN_POINT('Ctrl Pts',(101.633208512373,122.739705166155,44.2039215815208));
#21963=CARTESIAN_POINT('Ctrl Pts',(101.860867154298,122.385329399097,43.925862580649));
#21964=CARTESIAN_POINT('Ctrl Pts',(102.172129293686,122.245537374399,43.5934491246469));
#21965=CARTESIAN_POINT('Ctrl Pts',(102.369800991998,122.238070190751,43.3975371703006));
#21966=CARTESIAN_POINT('Ctrl Pts',(102.652462829699,122.238070190751,43.6801990080023));
#21967=CARTESIAN_POINT('Ctrl Pts',(102.456550875353,122.245537374399,43.8778707063143));
#21968=CARTESIAN_POINT('Ctrl Pts',(102.124137419351,122.385329399097,44.1891328457024));
#21969=CARTESIAN_POINT('Ctrl Pts',(101.846078418479,122.739705166155,44.4167914876269));
#21970=CARTESIAN_POINT('Ctrl Pts',(101.8,122.939812298928,44.45));
#21971=CARTESIAN_POINT('Ctrl Pts',(101.8,123.0375,44.45));
#21972=CARTESIAN_POINT('Ctrl Pts',(101.6,123.0375,44.25));
#21973=CARTESIAN_POINT('Ctrl Pts',(101.6,122.939812298928,44.25));
#21974=CARTESIAN_POINT('Ctrl Pts',(101.633208512373,122.739705166155,44.2039215815208));
#21975=CARTESIAN_POINT('Ctrl Pts',(101.860867154298,122.385329399097,43.925862580649));
#21976=CARTESIAN_POINT('Ctrl Pts',(102.172129293686,122.245537374399,43.5934491246469));
#21977=CARTESIAN_POINT('Ctrl Pts',(102.369800991998,122.238070190751,43.3975371703006));
#21978=CARTESIAN_POINT('Origin',(102.4,123.0375,-69.85));
#21979=CARTESIAN_POINT('',(101.6,123.0375,-69.85));
#21980=CARTESIAN_POINT('Origin',(101.6,122.2375,-107.95));
#21981=CARTESIAN_POINT('',(101.6,126.2,-69.85));
#21982=CARTESIAN_POINT('Origin',(102.4,126.2,-69.85));
#21983=CARTESIAN_POINT('',(102.4,127.,-69.85));
#21984=CARTESIAN_POINT('Origin',(120.65,126.2,43.65));
#21985=CARTESIAN_POINT('',(120.65,127.,43.65));
#21986=CARTESIAN_POINT('',(120.65,126.2,44.45));
#21987=CARTESIAN_POINT('Origin',(139.7,127.,-31.75));
#21988=CARTESIAN_POINT('Origin',(120.65,123.0375,43.65));
#21989=CARTESIAN_POINT('',(120.65,123.0375,44.45));
#21990=CARTESIAN_POINT('Origin',(101.6,122.2375,44.45));
#32281=UNCERTAINTY_MEASURE_WITH_UNIT(LENGTH_MEASURE(0.01),#32310,
'DISTANCE_ACCURACY_VALUE',
'Maximum model space distance between geometric entities at asserted c
onnectivities');
#32293=UNCERTAINTY_MEASURE_WITH_UNIT(LENGTH_MEASURE(0.01),#32310,
'DISTANCE_ACCURACY_VALUE',
'Maximum model space distance between geometric entities at asserted c
onnectivities');
#32297=(
GEOMETRIC_REPRESENTATION_CONTEXT(3)
GLOBAL_UNCERTAINTY_ASSIGNED_CONTEXT((#32281))
GLOBAL_UNIT_ASSIGNED_CONTEXT((#32310,#32312,#32313))
REPRESENTATION_CONTEXT('','3D')
);
#32309=(
GEOMETRIC_REPRESENTATION_CONTEXT(3)
GLOBAL_UNCERTAINTY_ASSIGNED_CONTEXT((#32293))
GLOBAL_UNIT_ASSIGNED_CONTEXT((#32310,#32312,#32313))
REPRESENTATION_CONTEXT('','3D')
);
#32310=(
LENGTH_UNIT()
NAMED_UNIT(*)
SI_UNIT(.MILLI.,.METRE.)
);
#32312=(
NAMED_UNIT(*)
PLANE_ANGLE_UNIT()
SI_UNIT($,.RADIAN.)
);
#32313=(
NAMED_UNIT(*)
SI_UNIT($,.STERADIAN.)
SOLID_ANGLE_UNIT()
);
#32317=SHAPE_DEFINITION_REPRESENTATION(#32332,#32364);
#32332=PRODUCT_DEFINITION_SHAPE('',$,#32380);
#32364=SHAPE_REPRESENTATION('',(#14095),#32297);
#32376=PRODUCT_DEFINITION_CONTEXT('part definition',#32423,'design');
#32380=PRODUCT_DEFINITION('2026-10-25-00-35-16-091',
'03_Outer_Door_Plate_3in',#32395,#32376);
#32395=PRODUCT_DEFINITION_FORMATION('',$,#32428);
#32423=APPLICATION_CONTEXT(
'Core Data for Automotive Mechanical Design Process');
#32424=PRODUCT_CONTEXT('part definition',#32423,'mechanical');
#32428=PRODUCT('2026-10-25-00-35-16-091','03_Outer_Door_Plate_3in',$,(#32424));
#32489=COLOUR_RGB('Sky Blue',0.24,0.69,0.87);
#32490=FILL_AREA_STYLE_COLOUR('',#32489);
#32491=FILL_AREA_STYLE('',(#32490));
#32492=SURFACE_STYLE_FILL_AREA(#32491);
#32493=SURFACE_SIDE_STYLE('',(#32492));
#32494=SURFACE_STYLE_USAGE(.BOTH.,#32493);
#32495=PRESENTATION_STYLE_ASSIGNMENT((#32494));
ENDSEC;
END-ISO-10303-21;
